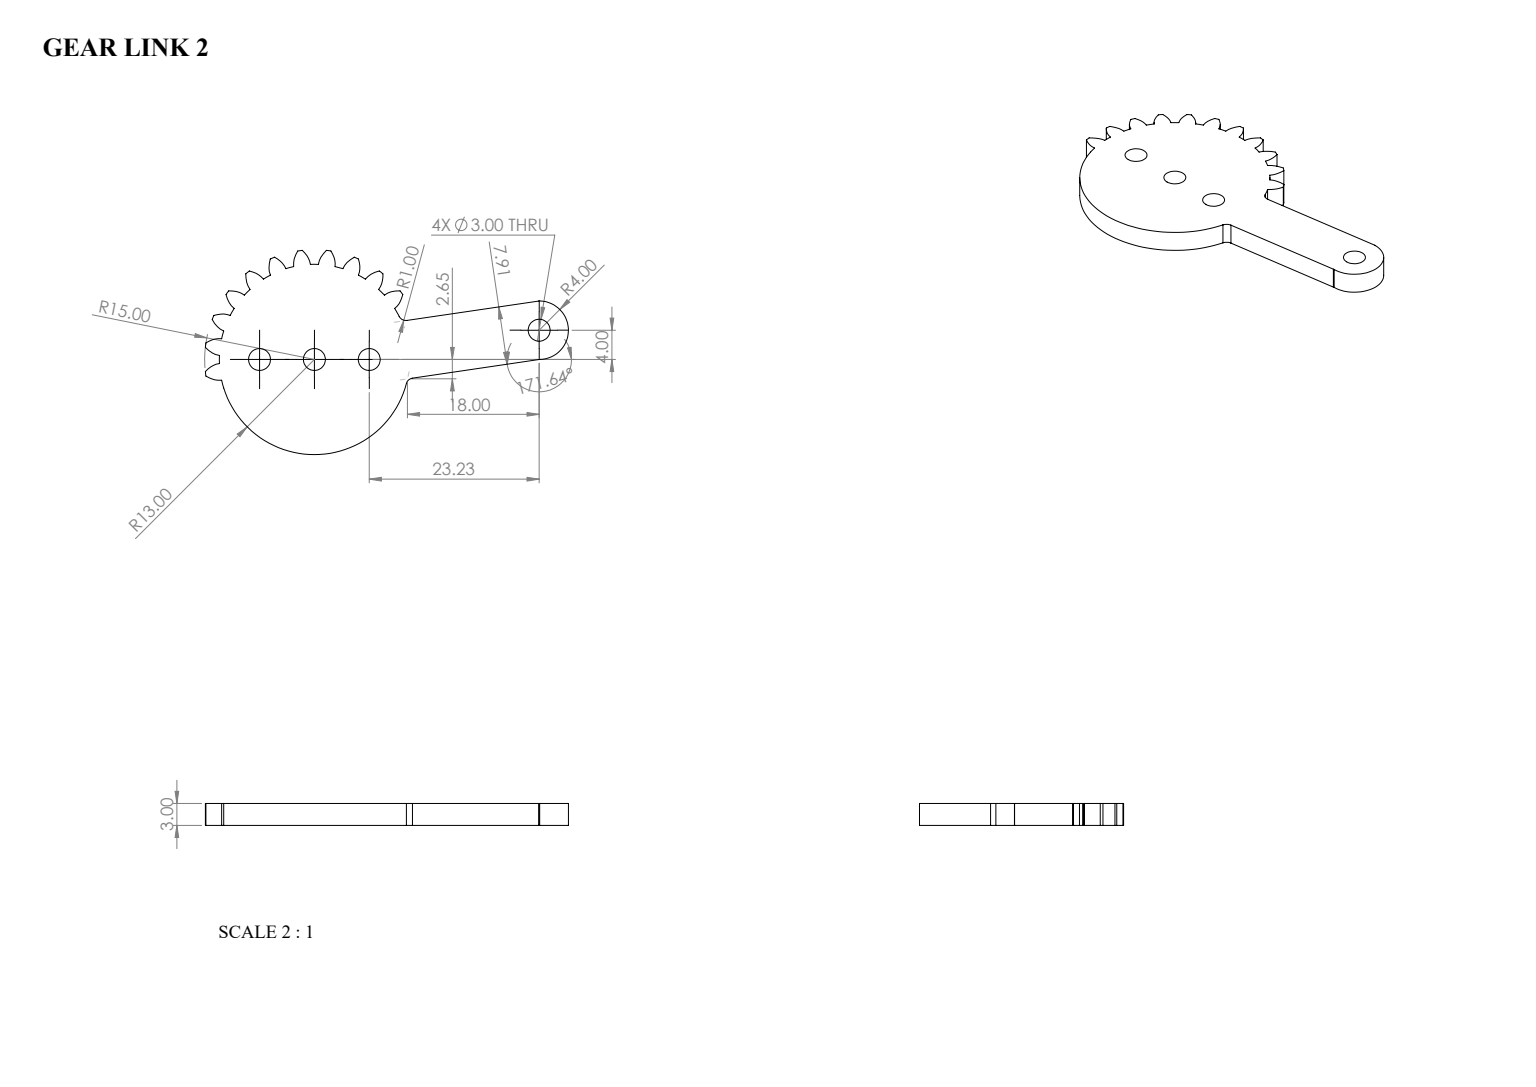
ISO-10303-21;
HEADER;
FILE_DESCRIPTION (('STEP AP214'),
    '1' );
FILE_NAME ('gear-link-2.step',
    '2026-10-11T23:18:24',
    ( '' ),
    ( '' ),
    'SwSTEP 2.0',
    'SolidWorks 2021',
    '' );
FILE_SCHEMA (( 'AUTOMOTIVE_DESIGN' ));
ENDSEC;

DATA;
#1=DIRECTION ( 'NONE',  ( 0.000000000000000000, 0.000000000000000000, -1.000000000000000000 ) ) ;
#3=ORIENTED_EDGE ( 'NONE', *, *, #624, .T. ) ;
#4=ORIENTED_EDGE ( 'NONE', *, *, #10369, .T. ) ;
#28=DIRECTION ( 'NONE',  ( 0.000000000000000000, 1.000000000000000000, 0.000000000000000000 ) ) ;
#34=CARTESIAN_POINT ( 'NONE',  ( 6.660877044263387781, 3.000000000000000000, -11.16999893002129696 ) ) ;
#42=EDGE_LOOP ( 'NONE', ( #11575, #10640, #9047, #10732 ) ) ;
#49=EDGE_CURVE ( 'NONE', #1339, #3948, #9205, .T. ) ;
#52=B_SPLINE_CURVE_WITH_KNOTS ( 'NONE', 3,
 ( #4525, #5550, #8714, #7882 ),
 .UNSPECIFIED., .F., .F.,
 ( 4, 4 ),
 ( 0.6363612417694253232, 0.6657793188270956231 ),
 .UNSPECIFIED. ) ;
#64=DIRECTION ( 'NONE',  ( 0.000000000000000000, 1.000000000000000000, 0.000000000000000000 ) ) ;
#73=LINE ( 'NONE', #7490, #793 ) ;
#82=B_SPLINE_SURFACE_WITH_KNOTS ( 'NONE', 2, 1, ( 
 ( #10714, #1415 ),
 ( #319, #8701 ),
 ( #12978, #11750 ) ),
 .UNSPECIFIED., .F., .F., .F.,
 ( 3, 3 ),
 ( 2, 2 ),
 ( 0.000000000000000000, 1.000000000000000000 ),
 ( 0.000000000000000000, 1.000000000000000000 ),
 .UNSPECIFIED. ) ;
#96=ORIENTED_EDGE ( 'NONE', *, *, #10741, .F. ) ;
#117=VERTEX_POINT ( 'NONE', #1849 ) ;
#127=CARTESIAN_POINT ( 'NONE',  ( -13.73660796332618261, 3.000000000000000000, -6.025412986832017204 ) ) ;
#132=ORIENTED_EDGE ( 'NONE', *, *, #11466, .T. ) ;
#134=DIRECTION ( 'NONE',  ( 0.000000000000000000, 0.000000000000000000, 1.000000000000000000 ) ) ;
#137=DIRECTION ( 'NONE',  ( 0.000000000000000000, 0.000000000000000000, -1.000000000000000000 ) ) ;
#144=VERTEX_POINT ( 'NONE', #5273 ) ;
#156=CARTESIAN_POINT ( 'NONE',  ( 0.5501230721522984979, 3.000000000000000000, -12.98835496148321766 ) ) ;
#157=CARTESIAN_POINT ( 'NONE',  ( -9.573149624528719315, 0.000000000000000000, -8.795158114916407754 ) ) ;
#160=ORIENTED_EDGE ( 'NONE', *, *, #10207, .F. ) ;
#161=ORIENTED_EDGE ( 'NONE', *, *, #7234, .F. ) ;
#162=B_SPLINE_SURFACE_WITH_KNOTS ( 'NONE', 3, 1, ( 
 ( #10319, #7359 ),
 ( #1025, #5084 ),
 ( #8312, #12538 ),
 ( #2123, #4325 ) ),
 .UNSPECIFIED., .F., .F., .F.,
 ( 4, 4 ),
 ( 2, 2 ),
 ( 0.000000000000000000, 0.5855695330273008592 ),
 ( 0.000000000000000000, 1.000000000000000000 ),
 .UNSPECIFIED. ) ;
#165=B_SPLINE_CURVE_WITH_KNOTS ( 'NONE', 3,
 ( #7734, #1615, #8698, #11948 ),
 .UNSPECIFIED., .F., .F.,
 ( 4, 4 ),
 ( 0.000000000000000000, 0.5855695330273008592 ),
 .UNSPECIFIED. ) ;
#166=ORIENTED_EDGE ( 'NONE', *, *, #10741, .T. ) ;
#168=DIRECTION ( 'NONE',  ( -0.000000000000000000, -1.000000000000000000, -0.000000000000000000 ) ) ;
#171=B_SPLINE_CURVE_WITH_KNOTS ( 'NONE', 3,
 ( #9035, #3811, #13254, #8012 ),
 .UNSPECIFIED., .F., .F.,
 ( 4, 4 ),
 ( 0.09090310649439187207, 0.1203211835519651524 ),
 .UNSPECIFIED. ) ;
#173=CARTESIAN_POINT ( 'NONE',  ( -8.795158114916672432, 3.000000000000000000, -9.573149624528774382 ) ) ;
#178=ORIENTED_EDGE ( 'NONE', *, *, #12277, .T. ) ;
#192=EDGE_CURVE ( 'NONE', #3774, #5500, #7308, .T. ) ;
#196=CARTESIAN_POINT ( 'NONE',  ( 13.40069634612381044, 0.000000000000000000, 2.546644602219900300 ) ) ;
#207=CARTESIAN_POINT ( 'NONE',  ( 12.08646469655232636, 3.000000000000000000, -8.883544964652022813 ) ) ;
#213=DIRECTION ( 'NONE',  ( 0.000000000000000000, 1.000000000000000000, 0.000000000000000000 ) ) ;
#215=CARTESIAN_POINT ( 'NONE',  ( -2.264806262022998062, 0.000000000000000000, -14.82803603298499340 ) ) ;
#218=ORIENTED_EDGE ( 'NONE', *, *, #842, .T. ) ;
#219=ORIENTED_EDGE ( 'NONE', *, *, #9373, .F. ) ;
#224=EDGE_CURVE ( 'NONE', #1339, #3538, #12385, .T. ) ;
#228=CARTESIAN_POINT ( 'NONE',  ( -13.52637830886122572, 3.000000000000000000, -2.928250210355275218 ) ) ;
#232=CARTESIAN_POINT ( 'NONE',  ( 2.928250210355320959, 3.000000000000000000, -13.52637830886121506 ) ) ;
#236=CARTESIAN_POINT ( 'NONE',  ( 6.970598036433451661, 3.000000000000000000, -10.97318381393796294 ) ) ;
#249=ORIENTED_EDGE ( 'NONE', *, *, #2547, .F. ) ;
#254=AXIS2_PLACEMENT_3D ( 'NONE', #5963, #13478, #3894 ) ;
#259=CARTESIAN_POINT ( 'NONE',  ( -6.970598036433426792, 3.000000000000000000, -10.97318381393771780 ) ) ;
#263=FACE_OUTER_BOUND ( 'NONE', #2351, .T. ) ;
#269=ORIENTED_EDGE ( 'NONE', *, *, #8193, .F. ) ;
#272=EDGE_LOOP ( 'NONE', ( #9491, #3874, #11052, #3338, #8276, #2839, #644, #11022, #10546, #6323, #4126, #5305, #5722, #5484, #10567, #12738, #3922, #6142, #1219, #3241, #11942, #4726, #6997, #1679, #13263, #12542, #5199, #9334, #7477, #1094, #5617, #8851, #4788, #11957, #10551, #9765, #5855, #13484, #4229, #12910, #8520, #970, #6174, #5838, #218, #6140, #7889, #11447, #8596, #13140, #12291, #13402, #12003, #12804 ) ) ;
#273=LINE ( 'NONE', #11625, #11249 ) ;
#274=CIRCLE ( 'NONE', #4001, 1.500000000000000222 ) ;
#276=B_SPLINE_SURFACE_WITH_KNOTS ( 'NONE', 3, 1, ( 
 ( #10127, #2687 ),
 ( #3651, #10063 ),
 ( #632, #13233 ),
 ( #12213, #10958 ) ),
 .UNSPECIFIED., .F., .F., .F.,
 ( 4, 4 ),
 ( 2, 2 ),
 ( 0.000000000000000000, 0.5855695330273008592 ),
 ( 0.000000000000000000, 1.000000000000000000 ),
 .UNSPECIFIED. ) ;
#281=CARTESIAN_POINT ( 'NONE',  ( 5.452638258930520010, 3.000000000000000000, -13.97385902380752754 ) ) ;
#288=VERTEX_POINT ( 'NONE', #5039 ) ;
#298=DIRECTION ( 'NONE',  ( -0.000000000000000000, -1.000000000000000000, -0.000000000000000000 ) ) ;
#300=FACE_BOUND ( 'NONE', #2086, .T. ) ;
#305=ORIENTED_EDGE ( 'NONE', *, *, #3885, .F. ) ;
#306=B_SPLINE_CURVE_WITH_KNOTS ( 'NONE', 3,
 ( #11706, #6473, #8390, #12616 ),
 .UNSPECIFIED., .F., .F.,
 ( 4, 4 ),
 ( 0.000000000000000000, 0.5855695330273008592 ),
 .UNSPECIFIED. ) ;
#315=LINE ( 'NONE', #6769, #11331 ) ;
#317=CARTESIAN_POINT ( 'NONE',  ( 1.650143266773734796, 0.000000000000000000, -14.90895795148410841 ) ) ;
#319=CARTESIAN_POINT ( 'NONE',  ( 5.741477348071313713, 3.000000000000000000, -13.86115248177180703 ) ) ;
#337=DIRECTION ( 'NONE',  ( -0.000000000000000000, -1.000000000000000000, -0.000000000000000000 ) ) ;
#360=LINE ( 'NONE', #3375, #1597 ) ;
#376=B_SPLINE_CURVE_WITH_KNOTS ( 'NONE', 2,
 ( #858, #13396, #4783 ),
 .UNSPECIFIED., .F., .F.,
 ( 3, 3 ),
 ( 0.000000000000000000, 1.000000000000000000 ),
 .UNSPECIFIED. ) ;
#385=ORIENTED_EDGE ( 'NONE', *, *, #12086, .T. ) ;
#390=CARTESIAN_POINT ( 'NONE',  ( 7.494008246337245716, 3.000000000000000000, -11.63517940784380578 ) ) ;
#391=CARTESIAN_POINT ( 'NONE',  ( -14.90895795148409420, 0.000000000000000000, 1.650143266773909101 ) ) ;
#395=CARTESIAN_POINT ( 'NONE',  ( -8.180229652970899323, 3.000000000000000000, -11.90209577080756276 ) ) ;
#406=B_SPLINE_CURVE_WITH_KNOTS ( 'NONE', 3,
 ( #3245, #11729, #7457, #5514 ),
 .UNSPECIFIED., .F., .F.,
 ( 4, 4 ),
 ( 0.1818127957067485756, 0.2112308727645026418 ),
 .UNSPECIFIED. ) ;
#411=DIRECTION ( 'NONE',  ( -0.000000000000000000, -1.000000000000000000, -0.000000000000000000 ) ) ;
#418=AXIS2_PLACEMENT_3D ( 'NONE', #13510, #5924, #10269 ) ;
#419=CARTESIAN_POINT ( 'NONE',  ( -14.90895795148411374, 0.000000000000000000, -1.650143266773683726 ) ) ;
#422=CARTESIAN_POINT ( 'NONE',  ( -5.452638258930639914, 3.000000000000000000, -13.97385902380748313 ) ) ;
#423=CARTESIAN_POINT ( 'NONE',  ( -13.52637830886122572, 0.000000000000000000, -2.928250210355275218 ) ) ;
#426=FACE_OUTER_BOUND ( 'NONE', #10907, .T. ) ;
#429=ADVANCED_FACE ( 'NONE', ( #4581 ), #2651, .F. ) ;
#430=ORIENTED_EDGE ( 'NONE', *, *, #1575, .F. ) ;
#438=CARTESIAN_POINT ( 'NONE',  ( 12.63269908545826503, 0.000000000000000000, -5.340493616518843467 ) ) ;
#448=EDGE_CURVE ( 'NONE', #3825, #117, #4011, .T. ) ;
#449=ORIENTED_EDGE ( 'NONE', *, *, #5832, .F. ) ;
#461=LINE ( 'NONE', #5837, #521 ) ;
#468=CARTESIAN_POINT ( 'NONE',  ( -0.1834773636644435324, 0.000000000000000000, -13.00394737445024873 ) ) ;
#473=CARTESIAN_POINT ( 'NONE',  ( 6.017756925049591921, 3.000000000000000000, -11.52330688609011844 ) ) ;
#483=CARTESIAN_POINT ( 'NONE',  ( -13.00394681030572208, 3.000000000000000000, -0.1834665838397169235 ) ) ;
#492=CARTESIAN_POINT ( 'NONE',  ( -2.830255545554292151, 3.000000000000000000, -12.68816982652971959 ) ) ;
#499=B_SPLINE_SURFACE_WITH_KNOTS ( 'NONE', 3, 1, ( 
 ( #6298, #5461 ),
 ( #3400, #5208 ),
 ( #10510, #11814 ),
 ( #1268, #10711 ) ),
 .UNSPECIFIED., .F., .F., .F.,
 ( 4, 4 ),
 ( 2, 2 ),
 ( 0.000000000000000000, 0.5855695330273008592 ),
 ( 0.000000000000000000, 1.000000000000000000 ),
 .UNSPECIFIED. ) ;
#501=ORIENTED_EDGE ( 'NONE', *, *, #4582, .F. ) ;
#502=ORIENTED_EDGE ( 'NONE', *, *, #9169, .T. ) ;
#511=CARTESIAN_POINT ( 'NONE',  ( -0.5501230721523990841, 0.000000000000000000, -12.98835496148299384 ) ) ;
#513=CARTESIAN_POINT ( 'NONE',  ( 8.883544964651964193, 3.000000000000000000, -12.08646469655236544 ) ) ;
#516=AXIS2_PLACEMENT_3D ( 'NONE', #8094, #8227, #869 ) ;
#520=ADVANCED_FACE ( 'NONE', ( #5381 ), #8916, .F. ) ;
#521=VECTOR ( 'NONE', #5626, 1000.000000000000000 ) ;
#522=B_SPLINE_CURVE_WITH_KNOTS ( 'NONE', 3,
 ( #12540, #2883, #11494, #4182 ),
 .UNSPECIFIED., .F., .F.,
 ( 4, 4 ),
 ( 0.000000000000000000, 0.5855695330273008592 ),
 .UNSPECIFIED. ) ;
#524=ORIENTED_EDGE ( 'NONE', *, *, #7234, .T. ) ;
#536=CARTESIAN_POINT ( 'NONE',  ( -11.90209577080766046, 3.000000000000000000, -8.180229652970757215 ) ) ;
#551=DIRECTION ( 'NONE',  ( -0.000000000000000000, -1.000000000000000000, -0.000000000000000000 ) ) ;
#556=CARTESIAN_POINT ( 'NONE',  ( -6.025412986832177076, 3.000000000000000000, -13.73660796332610268 ) ) ;
#557=ORIENTED_EDGE ( 'NONE', *, *, #3167, .F. ) ;
#565=EDGE_CURVE ( 'NONE', #13387, #8347, #11519, .T. ) ;
#567=ADVANCED_FACE ( 'NONE', ( #10952 ), #5726, .F. ) ;
#568=CARTESIAN_POINT ( 'NONE',  ( -11.52330688609014686, 0.000000000000000000, -6.017756925049552841 ) ) ;
#580=ORIENTED_EDGE ( 'NONE', *, *, #11985, .T. ) ;
#592=CARTESIAN_POINT ( 'NONE',  ( -3.893011711613112880, 0.000000000000000000, -12.40340517008282717 ) ) ;
#604=CARTESIAN_POINT ( 'NONE',  ( -12.68816982652970893, 3.000000000000000000, 2.830255545554337004 ) ) ;
#606=EDGE_LOOP ( 'NONE', ( #10674, #7647, #5644, #642 ) ) ;
#618=CARTESIAN_POINT ( 'NONE',  ( 13.40069634612381044, 3.000000000000000000, 2.546644602219900300 ) ) ;
#622=EDGE_LOOP ( 'NONE', ( #11651, #11442, #4299, #11608 ) ) ;
#623=LINE ( 'NONE', #3704, #12180 ) ;
#624=EDGE_CURVE ( 'NONE', #2462, #5247, #6615, .T. ) ;
#629=CARTESIAN_POINT ( 'NONE',  ( 12.08646469655232636, 3.000000000000000000, -8.883544964652022813 ) ) ;
#632=CARTESIAN_POINT ( 'NONE',  ( -6.329356821613726147, 3.000000000000000000, -12.30759122142001338 ) ) ;
#637=ORIENTED_EDGE ( 'NONE', *, *, #10382, .F. ) ;
#642=ORIENTED_EDGE ( 'NONE', *, *, #49, .T. ) ;
#644=ORIENTED_EDGE ( 'NONE', *, *, #13323, .T. ) ;
#670=ORIENTED_EDGE ( 'NONE', *, *, #4159, .T. ) ;
#678=EDGE_CURVE ( 'NONE', #6263, #3116, #360, .T. ) ;
#693=CARTESIAN_POINT ( 'NONE',  ( 6.329356821613516537, 3.000000000000000000, -12.30759122141987305 ) ) ;
#695=CARTESIAN_POINT ( 'NONE',  ( 3.893011711613070691, 0.000000000000000000, -12.40340517008307231 ) ) ;
#696=AXIS2_PLACEMENT_3D ( 'NONE', #10163, #9957, #13351 ) ;
#699=CARTESIAN_POINT ( 'NONE',  ( 30.82048254704846713, 0.000000000000000000, -7.998976482636475538 ) ) ;
#700=ADVANCED_FACE ( 'NONE', ( #10889 ), #9711, .F. ) ;
#701=LINE ( 'NONE', #3093, #9681 ) ;
#712=ORIENTED_EDGE ( 'NONE', *, *, #9478, .F. ) ;
#717=VECTOR ( 'NONE', #10109, 1000.000000000000000 ) ;
#721=CARTESIAN_POINT ( 'NONE',  ( -0.6724118135763151871, 0.000000000000000000, -13.82336506795071784 ) ) ;
#730=VECTOR ( 'NONE', #11828, 1000.000000000000000 ) ;
#746=VERTEX_POINT ( 'NONE', #7028 ) ;
#757=CARTESIAN_POINT ( 'NONE',  ( -11.70905276178463872, 3.000000000000000000, -9.375397774054366806 ) ) ;
#763=DIRECTION ( 'NONE',  ( 0.000000000000000000, 1.000000000000000000, 0.000000000000000000 ) ) ;
#772=AXIS2_PLACEMENT_3D ( 'NONE', #3729, #8758, #5667 ) ;
#776=CARTESIAN_POINT ( 'NONE',  ( -13.52637830886139092, 3.000000000000000000, 2.928250210355532790 ) ) ;
#777=( NAMED_UNIT ( * ) SI_UNIT ( $, .STERADIAN. ) SOLID_ANGLE_UNIT ( ) );
#786=EDGE_LOOP ( 'NONE', ( #2481, #7986, #11590, #10506 ) ) ;
#793=VECTOR ( 'NONE', #337, 1000.000000000000000 ) ;
#801=CARTESIAN_POINT ( 'NONE',  ( 10.97318381393774089, 3.000000000000000000, -6.970598036433387712 ) ) ;
#809=CARTESIAN_POINT ( 'NONE',  ( 30.73000000000000043, 0.000000000000000000, -3.999999999999999112 ) ) ;
#815=CARTESIAN_POINT ( 'NONE',  ( 0.000000000000000000, 3.000000000000000000, 0.000000000000000000 ) ) ;
#816=VERTEX_POINT ( 'NONE', #4965 ) ;
#819=ORIENTED_EDGE ( 'NONE', *, *, #11292, .T. ) ;
#827=CARTESIAN_POINT ( 'NONE',  ( -12.51336114795298471, 3.000000000000000000, -3.542894103880322998 ) ) ;
#836=B_SPLINE_CURVE_WITH_KNOTS ( 'NONE', 2,
 ( #3497, #5499, #8595 ),
 .UNSPECIFIED., .F., .F.,
 ( 3, 3 ),
 ( 0.000000000000000000, 1.000000000000000000 ),
 .UNSPECIFIED. ) ;
#838=DIRECTION ( 'NONE',  ( -0.000000000000000000, -1.000000000000000000, -0.000000000000000000 ) ) ;
#842=EDGE_CURVE ( 'NONE', #5225, #11316, #7958, .T. ) ;
#857=EDGE_CURVE ( 'NONE', #12351, #4567, #10437, .T. ) ;
#858=CARTESIAN_POINT ( 'NONE',  ( 6.025412986832064277, 0.000000000000000000, -13.73660796332615597 ) ) ;
#861=ORIENTED_EDGE ( 'NONE', *, *, #8629, .F. ) ;
#866=EDGE_CURVE ( 'NONE', #10985, #3576, #2838, .T. ) ;
#868=VERTEX_POINT ( 'NONE', #2820 ) ;
#869=DIRECTION ( 'NONE',  ( 0.000000000000000000, 0.000000000000000000, 1.000000000000000000 ) ) ;
#881=ORIENTED_EDGE ( 'NONE', *, *, #4007, .F. ) ;
#888=EDGE_CURVE ( 'NONE', #7605, #5310, #5227, .T. ) ;
#891=DIRECTION ( 'NONE',  ( -0.000000000000000000, -1.000000000000000000, -0.000000000000000000 ) ) ;
#899=VERTEX_POINT ( 'NONE', #2965 ) ;
#908=CARTESIAN_POINT ( 'NONE',  ( -13.97385902380755240, 0.000000000000000000, -5.452638258930474713 ) ) ;
#913=CARTESIAN_POINT ( 'NONE',  ( -4.821006024661084410, 3.000000000000000000, -13.61374091949017640 ) ) ;
#916=VERTEX_POINT ( 'NONE', #13435 ) ;
#926=DIRECTION ( 'NONE',  ( 0.000000000000000000, 0.000000000000000000, -1.000000000000000000 ) ) ;
#935=EDGE_CURVE ( 'NONE', #2130, #9763, #2355, .T. ) ;
#938=CARTESIAN_POINT ( 'NONE',  ( -11.90284147956865723, 0.000000000000000000, -9.133371500908332052 ) ) ;
#942=VECTOR ( 'NONE', #5646, 1000.000000000000000 ) ;
#953=VECTOR ( 'NONE', #5138, 1000.000000000000000 ) ;
#961=DIRECTION ( 'NONE',  ( -0.000000000000000000, -1.000000000000000000, -0.000000000000000000 ) ) ;
#966=ORIENTED_EDGE ( 'NONE', *, *, #7209, .T. ) ;
#970=ORIENTED_EDGE ( 'NONE', *, *, #8931, .T. ) ;
#973=CARTESIAN_POINT ( 'NONE',  ( -14.82803603298498629, 0.000000000000000000, 2.264806262023049577 ) ) ;
#974=CARTESIAN_POINT ( 'NONE',  ( 11.59535436762926430, 3.000000000000000000, -5.877734009726468756 ) ) ;
#981=AXIS2_PLACEMENT_3D ( 'NONE', #7760, #6861, #5625 ) ;
#990=CARTESIAN_POINT ( 'NONE',  ( 11.59535436762926430, 3.000000000000000000, -5.877734009726468756 ) ) ;
#999=FACE_OUTER_BOUND ( 'NONE', #9309, .T. ) ;
#1002=LINE ( 'NONE', #11939, #11502 ) ;
#1012=CARTESIAN_POINT ( 'NONE',  ( 30.65246752842885058, 3.000000000000000000, -7.988606140548566437 ) ) ;
#1014=COLOUR_RGB ( '',0.7803921568627451011, 0.7607843137254901578, 0.7411764705882353255 ) ;
#1015=EDGE_CURVE ( 'NONE', #1814, #11917, #3181, .T. ) ;
#1019=ORIENTED_EDGE ( 'NONE', *, *, #13582, .T. ) ;
#1025=CARTESIAN_POINT ( 'NONE',  ( 10.98198414889934682, 3.000000000000000000, -9.379342464487748998 ) ) ;
#1027=CARTESIAN_POINT ( 'NONE',  ( -11.52330688609014686, 0.000000000000000000, -6.017756925049552841 ) ) ;
#1029=EDGE_LOOP ( 'NONE', ( #6359, #8832, #10154, #3644 ) ) ;
#1031=ORIENTED_EDGE ( 'NONE', *, *, #12543, .T. ) ;
#1032=CARTESIAN_POINT ( 'NONE',  ( 0.1834774187694905023, 0.000000000000000000, -13.00394734430440025 ) ) ;
#1039=CARTESIAN_POINT ( 'NONE',  ( -9.379342464487789854, 3.000000000000000000, -10.98198414889931307 ) ) ;
#1040=B_SPLINE_CURVE_WITH_KNOTS ( 'NONE', 3,
 ( #2636, #10227, #3879, #8086 ),
 .UNSPECIFIED., .F., .F.,
 ( 4, 4 ),
 ( 0.000000000000000000, 0.5855695330273008592 ),
 .UNSPECIFIED. ) ;
#1048=CARTESIAN_POINT ( 'NONE',  ( -5.741477348071430065, 3.000000000000000000, -13.86115248177175374 ) ) ;
#1051=CARTESIAN_POINT ( 'NONE',  ( 1.133238802859644956, 3.000000000000000000, -14.39763212228013600 ) ) ;
#1069=CARTESIAN_POINT ( 'NONE',  ( -13.82336506795071607, 3.000000000000000000, 0.6724118135763649251 ) ) ;
#1083=CARTESIAN_POINT ( 'NONE',  ( 8.180229652970799847, 3.000000000000000000, -11.90209577080762848 ) ) ;
#1094=ORIENTED_EDGE ( 'NONE', *, *, #10459, .T. ) ;
#1099=CARTESIAN_POINT ( 'NONE',  ( 6.329356821613516537, 0.000000000000000000, -12.30759122141987305 ) ) ;
#1100=DIRECTION ( 'NONE',  ( 0.000000000000000000, 0.000000000000000000, 1.000000000000000000 ) ) ;
#1110=VERTEX_POINT ( 'NONE', #5486 ) ;
#1117=CARTESIAN_POINT ( 'NONE',  ( 30.66173999750687784, 0.000000000000000000, 0.01003121477750366919 ) ) ;
#1138=CARTESIAN_POINT ( 'NONE',  ( 11.70905276178455878, 3.000000000000000000, -9.375397774054460953 ) ) ;
#1140=CARTESIAN_POINT ( 'NONE',  ( 30.73000000000000043, 0.000000000000000000, -5.500000000000003553 ) ) ;
#1147=B_SPLINE_SURFACE_WITH_KNOTS ( 'NONE', 3, 1, ( 
 ( #8479, #9446 ),
 ( #12633, #11726 ),
 ( #8604, #11597 ),
 ( #6215, #2286 ) ),
 .UNSPECIFIED., .F., .F., .F.,
 ( 4, 4 ),
 ( 2, 2 ),
 ( 0.9090903094065657664, 0.9385083864668765097 ),
 ( 0.000000000000000000, 1.000000000000000000 ),
 .UNSPECIFIED. ) ;
#1157=DIRECTION ( 'NONE',  ( 0.000000000000000000, 1.000000000000000000, -0.000000000000000000 ) ) ;
#1173=CARTESIAN_POINT ( 'NONE',  ( -1.650143266773857142, 0.000000000000000000, -14.90895795148409952 ) ) ;
#1176=B_SPLINE_CURVE_WITH_KNOTS ( 'NONE', 3,
 ( #9855, #7659, #4562, #9597 ),
 .UNSPECIFIED., .F., .F.,
 ( 4, 4 ),
 ( 0.000000000000000000, 0.5855695330273008592 ),
 .UNSPECIFIED. ) ;
#1188=AXIS2_PLACEMENT_3D ( 'NONE', #809, #5000, #9194 ) ;
#1190=CARTESIAN_POINT ( 'NONE',  ( 9.299128225235451239, 3.000000000000000000, -10.25006213149493561 ) ) ;
#1195=LINE ( 'NONE', #173, #5307 ) ;
#1197=ORIENTED_EDGE ( 'NONE', *, *, #4427, .T. ) ;
#1206=ADVANCED_FACE ( 'NONE', ( #5426 ), #6831, .F. ) ;
#1214=CARTESIAN_POINT ( 'NONE',  ( 6.025412986832064277, 3.000000000000000000, -13.73660796332615597 ) ) ;
#1219=ORIENTED_EDGE ( 'NONE', *, *, #12818, .T. ) ;
#1221=ADVANCED_FACE ( 'NONE', ( #13141 ), #3750, .F. ) ;
#1228=CARTESIAN_POINT ( 'NONE',  ( -7.500000000000000000, 0.000000000000000000, 0.000000000000000000 ) ) ;
#1233=ORIENTED_EDGE ( 'NONE', *, *, #4398, .F. ) ;
#1238=CARTESIAN_POINT ( 'NONE',  ( 13.54609072798131209, 3.000000000000000000, 3.536018380791111415 ) ) ;
#1239=SURFACE_SIDE_STYLE ('',( #2602 ) ) ;
#1242=CARTESIAN_POINT ( 'NONE',  ( -1.958311002203252160, 3.000000000000000000, -14.87484884897975768 ) ) ;
#1245=ORIENTED_EDGE ( 'NONE', *, *, #13083, .F. ) ;
#1258=PLANE ( 'NONE',  #10858 ) ;
#1268=CARTESIAN_POINT ( 'NONE',  ( 6.025412986832064277, 3.000000000000000000, -13.73660796332615597 ) ) ;
#1269=EDGE_CURVE ( 'NONE', #9570, #11420, #3803, .T. ) ;
#1271=CARTESIAN_POINT ( 'NONE',  ( 1.133238802859644956, 0.000000000000000000, -14.39763212228013600 ) ) ;
#1272=CARTESIAN_POINT ( 'NONE',  ( -9.324917476840782982, 0.000000000000000000, -9.065441278446241924 ) ) ;
#1285=CARTESIAN_POINT ( 'NONE',  ( -6.660869762029062890, 3.000000000000000000, -11.17001010193236610 ) ) ;
#1286=B_SPLINE_CURVE_WITH_KNOTS ( 'NONE', 2,
 ( #7443, #4476, #6606 ),
 .UNSPECIFIED., .F., .F.,
 ( 3, 3 ),
 ( 0.000000000000000000, 1.000000000000000000 ),
 .UNSPECIFIED. ) ;
#1288=EDGE_CURVE ( 'NONE', #11402, #5247, #1374, .T. ) ;
#1300=LINE ( 'NONE', #2341, #8363 ) ;
#1305=CARTESIAN_POINT ( 'NONE',  ( -13.17831234185052836, 3.000000000000000000, -4.227250083625696320 ) ) ;
#1308=EDGE_LOOP ( 'NONE', ( #1538, #9293, #4547, #5125 ) ) ;
#1309=ORIENTED_EDGE ( 'NONE', *, *, #2939, .F. ) ;
#1310=CIRCLE ( 'NONE', #1531, 1.000000000000001776 ) ;
#1314=B_SPLINE_CURVE_WITH_KNOTS ( 'NONE', 2,
 ( #391, #12036, #6720 ),
 .UNSPECIFIED., .F., .F.,
 ( 3, 3 ),
 ( 0.000000000000000000, 1.000000000000000000 ),
 .UNSPECIFIED. ) ;
#1322=CARTESIAN_POINT ( 'NONE',  ( -7.500000000000000000, 3.000000000000000000, 1.500000000000000666 ) ) ;
#1326=ORIENTED_EDGE ( 'NONE', *, *, #3867, .F. ) ;
#1339=VERTEX_POINT ( 'NONE', #4111 ) ;
#1346=B_SPLINE_CURVE_WITH_KNOTS ( 'NONE', 3,
 ( #695, #4888, #9088, #13305 ),
 .UNSPECIFIED., .F., .F.,
 ( 4, 4 ),
 ( 0.7272709309819391787, 0.7566890080396341256 ),
 .UNSPECIFIED. ) ;
#1355=VECTOR ( 'NONE', #2270, 1000.000000000000000 ) ;
#1356=CARTESIAN_POINT ( 'NONE',  ( 2.631756770590782057, 0.000000000000000000, -14.20034848914875347 ) ) ;
#1359=EDGE_CURVE ( 'NONE', #11340, #1456, #10893, .T. ) ;
#1366=EDGE_CURVE ( 'NONE', #11919, #2149, #5640, .T. ) ;
#1369=FILL_AREA_STYLE_COLOUR ( '', #1014 ) ;
#1370=B_SPLINE_SURFACE_WITH_KNOTS ( 'NONE', 3, 1, ( 
 ( #5624, #9822 ),
 ( #536, #4591 ),
 ( #12042, #8847 ),
 ( #8776, #13068 ) ),
 .UNSPECIFIED., .F., .F., .F.,
 ( 4, 4 ),
 ( 2, 2 ),
 ( 0.000000000000000000, 0.5855695330273008592 ),
 ( 0.000000000000000000, 1.000000000000000000 ),
 .UNSPECIFIED. ) ;
#1374=B_SPLINE_CURVE_WITH_KNOTS ( 'NONE', 2,
 ( #2805, #7013, #1778 ),
 .UNSPECIFIED., .F., .F.,
 ( 3, 3 ),
 ( 0.000000000000000000, 1.000000000000000000 ),
 .UNSPECIFIED. ) ;
#1376=ORIENTED_EDGE ( 'NONE', *, *, #4336, .T. ) ;
#1382=ORIENTED_EDGE ( 'NONE', *, *, #1952, .F. ) ;
#1385=B_SPLINE_CURVE_WITH_KNOTS ( 'NONE', 3,
 ( #4618, #8805, #3586, #7305 ),
 .UNSPECIFIED., .F., .F.,
 ( 4, 4 ),
 ( 0.000000000000000000, 0.5855695330273008592 ),
 .UNSPECIFIED. ) ;
#1387=ORIENTED_EDGE ( 'NONE', *, *, #4398, .T. ) ;
#1388=CARTESIAN_POINT ( 'NONE',  ( -12.98835496148321944, 3.000000000000000000, -0.5501230721522550882 ) ) ;
#1393=CARTESIAN_POINT ( 'NONE',  ( -12.68816982652953840, 3.000000000000000000, -2.830255545554093644 ) ) ;
#1415=CARTESIAN_POINT ( 'NONE',  ( 6.025412986832064277, 0.000000000000000000, -13.73660796332615597 ) ) ;
#1416=DIRECTION ( 'NONE',  ( -0.000000000000000000, -1.000000000000000000, -0.000000000000000000 ) ) ;
#1428=CARTESIAN_POINT ( 'NONE',  ( 30.79786191028635400, 3.000000000000000000, -7.999232361977356653 ) ) ;
#1433=FACE_OUTER_BOUND ( 'NONE', #9405, .T. ) ;
#1436=ORIENTED_EDGE ( 'NONE', *, *, #1948, .F. ) ;
#1439=ORIENTED_EDGE ( 'NONE', *, *, #8319, .F. ) ;
#1441=VERTEX_POINT ( 'NONE', #1624 ) ;
#1456=VERTEX_POINT ( 'NONE', #592 ) ;
#1467=FACE_BOUND ( 'NONE', #10598, .T. ) ;
#1468=CARTESIAN_POINT ( 'NONE',  ( -12.68816982652953840, 3.000000000000000000, -2.830255545554093644 ) ) ;
#1480=CARTESIAN_POINT ( 'NONE',  ( 0.5501230721522984979, 0.000000000000000000, -12.98835496148321766 ) ) ;
#1486=B_SPLINE_SURFACE_WITH_KNOTS ( 'NONE', 3, 1, ( 
 ( #8264, #973 ),
 ( #9432, #4193 ),
 ( #776, #4969 ),
 ( #13377, #9164 ) ),
 .UNSPECIFIED., .F., .F., .F.,
 ( 4, 4 ),
 ( 2, 2 ),
 ( 0.000000000000000000, 0.5855695330273008592 ),
 ( 0.000000000000000000, 1.000000000000000000 ),
 .UNSPECIFIED. ) ;
#1504=EDGE_LOOP ( 'NONE', ( #1890, #2339, #249, #3 ) ) ;
#1517=CARTESIAN_POINT ( 'NONE',  ( -13.00394681030572208, 0.000000000000000000, -0.1834665838397169235 ) ) ;
#1524=B_SPLINE_CURVE_WITH_KNOTS ( 'NONE', 3,
 ( #12864, #7682, #390, #9619 ),
 .UNSPECIFIED., .F., .F.,
 ( 4, 4 ),
 ( 0.000000000000000000, 0.5855695330273008592 ),
 .UNSPECIFIED. ) ;
#1529=CARTESIAN_POINT ( 'NONE',  ( 9.065480927540312095, 0.000000000000000000, -9.324856600128422102 ) ) ;
#1531=AXIS2_PLACEMENT_3D ( 'NONE', #1238, #4264, #5428 ) ;
#1533=ORIENTED_EDGE ( 'NONE', *, *, #12497, .F. ) ;
#1536=VERTEX_POINT ( 'NONE', #7032 ) ;
#1537=EDGE_CURVE ( 'NONE', #13428, #13474, #4113, .T. ) ;
#1538=ORIENTED_EDGE ( 'NONE', *, *, #12078, .T. ) ;
#1553=ORIENTED_EDGE ( 'NONE', *, *, #10207, .T. ) ;
#1558=CARTESIAN_POINT ( 'NONE',  ( -1.650143266773857142, 0.000000000000000000, -14.90895795148409952 ) ) ;
#1566=CARTESIAN_POINT ( 'NONE',  ( -13.61374091949023679, 3.000000000000000000, -4.821006024660923650 ) ) ;
#1568=AXIS2_PLACEMENT_3D ( 'NONE', #12469, #12655, #8432 ) ;
#1570=ORIENTED_EDGE ( 'NONE', *, *, #2217, .F. ) ;
#1575=EDGE_CURVE ( 'NONE', #6867, #8751, #9965, .T. ) ;
#1582=FACE_OUTER_BOUND ( 'NONE', #2814, .T. ) ;
#1593=FACE_OUTER_BOUND ( 'NONE', #5258, .T. ) ;
#1597=VECTOR ( 'NONE', #7587, 1000.000000000000000 ) ;
#1608=VERTEX_POINT ( 'NONE', #10196 ) ;
#1609=ORIENTED_EDGE ( 'NONE', *, *, #2578, .F. ) ;
#1615=CARTESIAN_POINT ( 'NONE',  ( 10.98198414889934682, 0.000000000000000000, -9.379342464487748998 ) ) ;
#1619=CARTESIAN_POINT ( 'NONE',  ( -9.065441275458884007, 0.000000000000000000, -9.324917484779556176 ) ) ;
#1623=VECTOR ( 'NONE', #2118, 1000.000000000000000 ) ;
#1624=CARTESIAN_POINT ( 'NONE',  ( 8.795158114916441505, 3.000000000000000000, -9.573149624528689117 ) ) ;
#1627=AXIS2_PLACEMENT_3D ( 'NONE', #11632, #9626, #8578 ) ;
#1638=EDGE_CURVE ( 'NONE', #12749, #2659, #1346, .T. ) ;
#1640=CARTESIAN_POINT ( 'NONE',  ( -2.830255545554292151, 3.000000000000000000, -12.68816982652971959 ) ) ;
#1648=EDGE_LOOP ( 'NONE', ( #5645, #712, #3236, #11092 ) ) ;
#1651=VERTEX_POINT ( 'NONE', #9558 ) ;
#1654=VECTOR ( 'NONE', #5931, 1000.000000000000000 ) ;
#1661=ORIENTED_EDGE ( 'NONE', *, *, #2538, .F. ) ;
#1679=ORIENTED_EDGE ( 'NONE', *, *, #5232, .T. ) ;
#1680=ORIENTED_EDGE ( 'NONE', *, *, #6158, .F. ) ;
#1693=CARTESIAN_POINT ( 'NONE',  ( -3.893011711613112880, 3.000000000000000000, -12.40340517008282717 ) ) ;
#1695=DIRECTION ( 'NONE',  ( 0.000000000000000000, 1.000000000000000000, -0.000000000000000000 ) ) ;
#1696=ORIENTED_EDGE ( 'NONE', *, *, #4159, .F. ) ;
#1702=CARTESIAN_POINT ( 'NONE',  ( -6.970598036433426792, 0.000000000000000000, -10.97318381393771780 ) ) ;
#1705=ADVANCED_FACE ( 'NONE', ( #8638 ), #3873, .F. ) ;
#1716=EDGE_CURVE ( 'NONE', #8003, #11262, #1524, .T. ) ;
#1718=DIRECTION ( 'NONE',  ( -0.000000000000000000, -1.000000000000000000, -0.000000000000000000 ) ) ;
#1722=CARTESIAN_POINT ( 'NONE',  ( -14.90895795148411374, 3.000000000000000000, -1.650143266773683726 ) ) ;
#1726=ORIENTED_EDGE ( 'NONE', *, *, #7893, .F. ) ;
#1731=CARTESIAN_POINT ( 'NONE',  ( 6.025412986832064277, 3.000000000000000000, -13.73660796332615597 ) ) ;
#1741=CARTESIAN_POINT ( 'NONE',  ( -12.40340517008309185, 3.000000000000000000, -3.893011711613028947 ) ) ;
#1748=ORIENTED_EDGE ( 'NONE', *, *, #9633, .T. ) ;
#1749=CARTESIAN_POINT ( 'NONE',  ( -6.025412986832177076, 3.000000000000000000, -13.73660796332610268 ) ) ;
#1751=CARTESIAN_POINT ( 'NONE',  ( -7.494008246337227952, 0.000000000000000000, -11.63517940784355886 ) ) ;
#1762=ORIENTED_EDGE ( 'NONE', *, *, #13322, .F. ) ;
#1769=CARTESIAN_POINT ( 'NONE',  ( 6.343080161942737938, 0.000000000000000000, -11.35348358516942469 ) ) ;
#1771=CARTESIAN_POINT ( 'NONE',  ( -14.82803603298498629, 3.000000000000000000, 2.264806262023049577 ) ) ;
#1772=ADVANCED_FACE ( 'NONE', ( #5348 ), #4522, .F. ) ;
#1778=CARTESIAN_POINT ( 'NONE',  ( 1.650143266773734796, 0.000000000000000000, -14.90895795148410841 ) ) ;
#1787=VECTOR ( 'NONE', #5884, 1000.000000000000000 ) ;
#1795=ORIENTED_EDGE ( 'NONE', *, *, #6353, .F. ) ;
#1814=VERTEX_POINT ( 'NONE', #1558 ) ;
#1822=VECTOR ( 'NONE', #2673, 1000.000000000000000 ) ;
#1830=CARTESIAN_POINT ( 'NONE',  ( -0.6724118135763151871, 3.000000000000000000, -13.82336506795071784 ) ) ;
#1837=ORIENTED_EDGE ( 'NONE', *, *, #5832, .T. ) ;
#1842=CARTESIAN_POINT ( 'NONE',  ( -8.795158114916672432, 3.000000000000000000, -9.573149624528774382 ) ) ;
#1849=CARTESIAN_POINT ( 'NONE',  ( 12.57851281883977457, 3.000000000000000000, 3.283445639306028063 ) ) ;
#1853=EDGE_LOOP ( 'NONE', ( #6961, #4497, #1680, #7692 ) ) ;
#1854=EDGE_CURVE ( 'NONE', #6430, #6340, #12989, .T. ) ;
#1870=ORIENTED_EDGE ( 'NONE', *, *, #9876, .T. ) ;
#1883=DIRECTION ( 'NONE',  ( -0.000000000000000000, -1.000000000000000000, -0.000000000000000000 ) ) ;
#1886=VECTOR ( 'NONE', #961, 1000.000000000000000 ) ;
#1890=ORIENTED_EDGE ( 'NONE', *, *, #10284, .T. ) ;
#1894=AXIS2_PLACEMENT_3D ( 'NONE', #10392, #13498, #1 ) ;
#1895=CARTESIAN_POINT ( 'NONE',  ( 10.98198414889934682, 3.000000000000000000, -9.379342464487748998 ) ) ;
#1907=PRODUCT_DEFINITION_FORMATION_WITH_SPECIFIED_SOURCE ( 'ANY', '', #7531, .NOT_KNOWN. ) ;
#1908=ORIENTED_EDGE ( 'NONE', *, *, #8249, .T. ) ;
#1915=B_SPLINE_SURFACE_WITH_KNOTS ( 'NONE', 3, 1, ( 
 ( #3445, #568 ),
 ( #13165, #2685 ),
 ( #6890, #7654 ),
 ( #11857, #2416 ) ),
 .UNSPECIFIED., .F., .F., .F.,
 ( 4, 4 ),
 ( 2, 2 ),
 ( 0.000000000000000000, 0.5855695330273008592 ),
 ( 0.000000000000000000, 1.000000000000000000 ),
 .UNSPECIFIED. ) ;
#1916=CARTESIAN_POINT ( 'NONE',  ( -14.87484884897975057, 3.000000000000000000, 1.958311002203303453 ) ) ;
#1921=ORIENTED_EDGE ( 'NONE', *, *, #9861, .T. ) ;
#1923=CARTESIAN_POINT ( 'NONE',  ( -3.188443695493920593, 0.000000000000000000, -12.60833606734848189 ) ) ;
#1929=CARTESIAN_POINT ( 'NONE',  ( -12.60833596047604210, 0.000000000000000000, -3.188441730140805674 ) ) ;
#1939=FACE_OUTER_BOUND ( 'NONE', #12013, .T. ) ;
#1941=CARTESIAN_POINT ( 'NONE',  ( 1.650143266773734796, 0.000000000000000000, -14.90895795148410841 ) ) ;
#1948=EDGE_CURVE ( 'NONE', #3825, #916, #12465, .T. ) ;
#1952=EDGE_CURVE ( 'NONE', #12534, #13401, #6453, .T. ) ;
#1958=LINE ( 'NONE', #13534, #11523 ) ;
#1961=CARTESIAN_POINT ( 'NONE',  ( -14.90895795148409420, 3.000000000000000000, 1.650143266773909101 ) ) ;
#1970=EDGE_CURVE ( 'NONE', #3576, #11919, #6278, .T. ) ;
#1972=CARTESIAN_POINT ( 'NONE',  ( -3.188443695493920593, 3.000000000000000000, -12.60833606734848189 ) ) ;
#1974=DIRECTION ( 'NONE',  ( -0.000000000000000000, -1.000000000000000000, -0.000000000000000000 ) ) ;
#1975=LINE ( 'NONE', #1012, #7945 ) ;
#1992=CARTESIAN_POINT ( 'NONE',  ( 30.73000000000000043, 3.000000000000000000, -2.499999999999995115 ) ) ;
#2001=CYLINDRICAL_SURFACE ( 'NONE', #418, 3.999999999999997335 ) ;
#2007=FACE_OUTER_BOUND ( 'NONE', #1504, .T. ) ;
#2010=ORIENTED_EDGE ( 'NONE', *, *, #7467, .F. ) ;
#2014=CARTESIAN_POINT ( 'NONE',  ( -5.741477348071430065, 0.000000000000000000, -13.86115248177175374 ) ) ;
#2020=CARTESIAN_POINT ( 'NONE',  ( -10.97318381393799136, 0.000000000000000000, -6.970598036433411693 ) ) ;
#2025=DIRECTION ( 'NONE',  ( -0.000000000000000000, -1.000000000000000000, -0.000000000000000000 ) ) ;
#2039=ADVANCED_FACE ( 'NONE', ( #2857 ), #6234, .F. ) ;
#2043=CARTESIAN_POINT ( 'NONE',  ( 6.970598036433451661, 0.000000000000000000, -10.97318381393796294 ) ) ;
#2045=EDGE_CURVE ( 'NONE', #4765, #7515, #2995, .T. ) ;
#2069=CARTESIAN_POINT ( 'NONE',  ( -0.1834773636644435324, 0.000000000000000000, -13.00394737445024873 ) ) ;
#2070=ORIENTED_EDGE ( 'NONE', *, *, #4899, .T. ) ;
#2078=CARTESIAN_POINT ( 'NONE',  ( -12.56843238770841786, 3.000000000000000000, 3.367671042046304741 ) ) ;
#2079=CARTESIAN_POINT ( 'NONE',  ( 1.650143266773734796, 3.000000000000000000, -14.90895795148410841 ) ) ;
#2086=EDGE_LOOP ( 'NONE', ( #3854, #8076 ) ) ;
#2095=CARTESIAN_POINT ( 'NONE',  ( 12.08646469655232636, 3.000000000000000000, -8.883544964652022813 ) ) ;
#2101=EDGE_CURVE ( 'NONE', #6340, #9161, #7137, .T. ) ;
#2113=ORIENTED_EDGE ( 'NONE', *, *, #1970, .F. ) ;
#2114=EDGE_CURVE ( 'NONE', #117, #4831, #9542, .T. ) ;
#2118=DIRECTION ( 'NONE',  ( -0.000000000000000000, -1.000000000000000000, -0.000000000000000000 ) ) ;
#2123=CARTESIAN_POINT ( 'NONE',  ( 9.573149624528804580, 3.000000000000000000, -8.795158114916638681 ) ) ;
#2124=CARTESIAN_POINT ( 'NONE',  ( -12.68816982652953840, 3.000000000000000000, -2.830255545554093644 ) ) ;
#2125=CARTESIAN_POINT ( 'NONE',  ( -10.97318381393799136, 3.000000000000000000, -6.970598036433411693 ) ) ;
#2127=ADVANCED_FACE ( 'NONE', ( #11745 ), #6083, .F. ) ;
#2130=VERTEX_POINT ( 'NONE', #10710 ) ;
#2135=B_SPLINE_SURFACE_WITH_KNOTS ( 'NONE', 3, 1, ( 
 ( #4543, #6477 ),
 ( #10613, #10685 ),
 ( #1305, #9641 ),
 ( #4406, #6682 ) ),
 .UNSPECIFIED., .F., .F., .F.,
 ( 4, 4 ),
 ( 2, 2 ),
 ( 0.000000000000000000, 0.5855695330273008592 ),
 ( 0.000000000000000000, 1.000000000000000000 ),
 .UNSPECIFIED. ) ;
#2143=ORIENTED_EDGE ( 'NONE', *, *, #7450, .T. ) ;
#2146=ORIENTED_EDGE ( 'NONE', *, *, #9861, .F. ) ;
#2149=VERTEX_POINT ( 'NONE', #4303 ) ;
#2158=CARTESIAN_POINT ( 'NONE',  ( 13.54609072798131209, 3.000000000000000000, 3.536018380791111415 ) ) ;
#2162=ORIENTED_EDGE ( 'NONE', *, *, #12261, .F. ) ;
#2167=CARTESIAN_POINT ( 'NONE',  ( -14.90895795148409420, 0.000000000000000000, 1.650143266773909101 ) ) ;
#2173=B_SPLINE_CURVE_WITH_KNOTS ( 'NONE', 3,
 ( #11816, #8826, #13050, #2579 ),
 .UNSPECIFIED., .F., .F.,
 ( 4, 4 ),
 ( 0.000000000000000000, 0.5855695330273008592 ),
 .UNSPECIFIED. ) ;
#2174=DIRECTION ( 'NONE',  ( 0.000000000000000000, 1.000000000000000000, -0.000000000000000000 ) ) ;
#2179=CARTESIAN_POINT ( 'NONE',  ( -14.82803603298502360, 0.000000000000000000, -2.264806262022826644 ) ) ;
#2181=CARTESIAN_POINT ( 'NONE',  ( 7.494008246337245716, 0.000000000000000000, -11.63517940784380578 ) ) ;
#2189=ORIENTED_EDGE ( 'NONE', *, *, #12522, .F. ) ;
#2202=DIRECTION ( 'NONE',  ( 0.000000000000000000, 0.000000000000000000, 1.000000000000000000 ) ) ;
#2209=ORIENTED_EDGE ( 'NONE', *, *, #5475, .F. ) ;
#2210=CARTESIAN_POINT ( 'NONE',  ( -6.025412986832177076, 3.000000000000000000, -13.73660796332610268 ) ) ;
#2217=EDGE_CURVE ( 'NONE', #11316, #11354, #9554, .T. ) ;
#2220=CARTESIAN_POINT ( 'NONE',  ( 2.264806262022877714, 0.000000000000000000, -14.82803603298501471 ) ) ;
#2222=CARTESIAN_POINT ( 'NONE',  ( -9.573149624528719315, 3.000000000000000000, -8.795158114916407754 ) ) ;
#2234=LINE ( 'NONE', #10653, #9228 ) ;
#2235=CARTESIAN_POINT ( 'NONE',  ( -11.90284147956865723, 0.000000000000000000, -9.133371500908332052 ) ) ;
#2236=B_SPLINE_CURVE_WITH_KNOTS ( 'NONE', 3,
 ( #12874, #3419, #5556, #3153 ),
 .UNSPECIFIED., .F., .F.,
 ( 4, 4 ),
 ( 0.000000000000000000, 0.5855695330273008592 ),
 .UNSPECIFIED. ) ;
#2237=CARTESIAN_POINT ( 'NONE',  ( 30.79786191028635400, 3.000000000000000000, -6.999232361977355765 ) ) ;
#2251=CARTESIAN_POINT ( 'NONE',  ( 2.264806262022877714, 0.000000000000000000, -14.82803603298501471 ) ) ;
#2262=CARTESIAN_POINT ( 'NONE',  ( 9.573149624528804580, 3.000000000000000000, -8.795158114916638681 ) ) ;
#2267=CARTESIAN_POINT ( 'NONE',  ( 13.54609072798131209, 0.000000000000000000, 3.536018380791111415 ) ) ;
#2270=DIRECTION ( 'NONE',  ( -0.000000000000000000, -1.000000000000000000, -0.000000000000000000 ) ) ;
#2274=ORIENTED_EDGE ( 'NONE', *, *, #1537, .F. ) ;
#2281=VECTOR ( 'NONE', #9666, 1000.000000000000000 ) ;
#2284=DIRECTION ( 'NONE',  ( 0.9893737785712105604, -0.000000000000000000, -0.1453943818575020863 ) ) ;
#2286=CARTESIAN_POINT ( 'NONE',  ( 8.795158114916441505, 0.000000000000000000, -9.573149624528689117 ) ) ;
#2288=DIRECTION ( 'NONE',  ( -0.000000000000000000, -1.000000000000000000, -0.000000000000000000 ) ) ;
#2290=CARTESIAN_POINT ( 'NONE',  ( 6.343080161942737938, 3.000000000000000000, -11.35348358516942469 ) ) ;
#2296=CARTESIAN_POINT ( 'NONE',  ( 6.660877044263387781, 0.000000000000000000, -11.16999893002129696 ) ) ;
#2298=B_SPLINE_CURVE_WITH_KNOTS ( 'NONE', 3,
 ( #10242, #13270, #3829, #10304 ),
 .UNSPECIFIED., .F., .F.,
 ( 4, 4 ),
 ( 0.000000000000000000, 0.5855695330273008592 ),
 .UNSPECIFIED. ) ;
#2303=ORIENTED_EDGE ( 'NONE', *, *, #9275, .F. ) ;
#2305=B_SPLINE_CURVE_WITH_KNOTS ( 'NONE', 3,
 ( #6119, #2807, #7016, #9208 ),
 .UNSPECIFIED., .F., .F.,
 ( 4, 4 ),
 ( 0.000000000000000000, 0.5855695330273008592 ),
 .UNSPECIFIED. ) ;
#2306=CARTESIAN_POINT ( 'NONE',  ( -13.82336506795071607, 0.000000000000000000, 0.6724118135763649251 ) ) ;
#2313=CARTESIAN_POINT ( 'NONE',  ( -1.650143266773857142, 3.000000000000000000, -14.90895795148409952 ) ) ;
#2317=VECTOR ( 'NONE', #168, 1000.000000000000000 ) ;
#2318=CIRCLE ( 'NONE', #1894, 1.000000000000000888 ) ;
#2325=B_SPLINE_CURVE_WITH_KNOTS ( 'NONE', 3,
 ( #9684, #11969, #12932, #10927 ),
 .UNSPECIFIED., .F., .F.,
 ( 4, 4 ),
 ( 0.000000000000000000, 0.5855695330273008592 ),
 .UNSPECIFIED. ) ;
#2329=CARTESIAN_POINT ( 'NONE',  ( -6.343077614891082128, 3.000000000000000000, -11.35348748332310720 ) ) ;
#2330=CARTESIAN_POINT ( 'NONE',  ( -13.86115248177182835, 0.000000000000000000, -5.741477348071267528 ) ) ;
#2339=ORIENTED_EDGE ( 'NONE', *, *, #7209, .F. ) ;
#2341=CARTESIAN_POINT ( 'NONE',  ( 30.82048254704846713, 3.000000000000000000, -7.998976482636475538 ) ) ;
#2343=DIRECTION ( 'NONE',  ( 0.000000000000000000, 0.000000000000000000, -1.000000000000000000 ) ) ;
#2351=EDGE_LOOP ( 'NONE', ( #6981, #2596, #6036, #2146 ) ) ;
#2352=CARTESIAN_POINT ( 'NONE',  ( -13.00394572736061605, 0.000000000000000000, 0.1835083749157108701 ) ) ;
#2355=B_SPLINE_CURVE_WITH_KNOTS ( 'NONE', 3,
 ( #7300, #1032, #2069, #9426 ),
 .UNSPECIFIED., .F., .F.,
 ( 4, 4 ),
 ( 0.6363612417694253232, 0.6657793188270956231 ),
 .UNSPECIFIED. ) ;
#2359=CARTESIAN_POINT ( 'NONE',  ( -8.883544964652065445, 3.000000000000000000, -12.08646469655229438 ) ) ;
#2366=CARTESIAN_POINT ( 'NONE',  ( 6.343080161942737938, 0.000000000000000000, -11.35348358516942469 ) ) ;
#2376=CARTESIAN_POINT ( 'NONE',  ( -11.70905276178463872, 3.000000000000000000, -9.375397774054366806 ) ) ;
#2380=VERTEX_POINT ( 'NONE', #4010 ) ;
#2398=CARTESIAN_POINT ( 'NONE',  ( 12.08646469655232636, 0.000000000000000000, -8.883544964652022813 ) ) ;
#2401=( NAMED_UNIT ( * ) SI_UNIT ( $, .STERADIAN. ) SOLID_ANGLE_UNIT ( ) );
#2412=ORIENTED_EDGE ( 'NONE', *, *, #5232, .F. ) ;
#2413=DIRECTION ( 'NONE',  ( 0.9893737785712105604, 0.000000000000000000, -0.1453943818575021141 ) ) ;
#2416=CARTESIAN_POINT ( 'NONE',  ( -13.73660796332618261, 0.000000000000000000, -6.025412986832017204 ) ) ;
#2419=DIRECTION ( 'NONE',  ( 0.000000000000000000, 0.000000000000000000, 1.000000000000000000 ) ) ;
#2426=VERTEX_POINT ( 'NONE', #12443 ) ;
#2434=ADVANCED_BREP_SHAPE_REPRESENTATION ( '', ( #4005, #10007 ), #6949 ) ;
#2444=CARTESIAN_POINT ( 'NONE',  ( 4.821006024660968947, 3.000000000000000000, -13.61374091949021015 ) ) ;
#2448=VERTEX_POINT ( 'NONE', #1749 ) ;
#2462=VERTEX_POINT ( 'NONE', #13529 ) ;
#2470=( NAMED_UNIT ( * ) SI_UNIT ( $, .STERADIAN. ) SOLID_ANGLE_UNIT ( ) );
#2471=B_SPLINE_SURFACE_WITH_KNOTS ( 'NONE', 3, 1, ( 
 ( #8433, #8498 ),
 ( #3851, #3981 ),
 ( #8116, #11365 ),
 ( #5018, #2958 ) ),
 .UNSPECIFIED., .F., .F., .F.,
 ( 4, 4 ),
 ( 2, 2 ),
 ( 0.7272709309819391787, 0.7566890080396341256 ),
 ( 0.000000000000000000, 1.000000000000000000 ),
 .UNSPECIFIED. ) ;
#2473=CARTESIAN_POINT ( 'NONE',  ( -10.25006213149496936, 3.000000000000000000, -9.299128225235415712 ) ) ;
#2481=ORIENTED_EDGE ( 'NONE', *, *, #3216, .T. ) ;
#2483=EDGE_CURVE ( 'NONE', #3948, #9570, #10881, .T. ) ;
#2495=CARTESIAN_POINT ( 'NONE',  ( -12.68816982652970893, 0.000000000000000000, 2.830255545554337004 ) ) ;
#2498=EDGE_LOOP ( 'NONE', ( #9710, #6063, #1921, #7432 ) ) ;
#2512=FACE_OUTER_BOUND ( 'NONE', #7420, .T. ) ;
#2516=EDGE_CURVE ( 'NONE', #1441, #816, #11183, .T. ) ;
#2519=VECTOR ( 'NONE', #11293, 1000.000000000000000 ) ;
#2523=CARTESIAN_POINT ( 'NONE',  ( -6.017756925049793537, 3.000000000000000000, -11.52330688609026232 ) ) ;
#2536=EDGE_LOOP ( 'NONE', ( #10265, #6533, #1609, #3765 ) ) ;
#2538=EDGE_CURVE ( 'NONE', #11094, #10001, #5591, .T. ) ;
#2541=AXIS2_PLACEMENT_3D ( 'NONE', #9215, #7296, #13427 ) ;
#2547=EDGE_CURVE ( 'NONE', #2462, #13403, #13162, .T. ) ;
#2550=ORIENTED_EDGE ( 'NONE', *, *, #1716, .F. ) ;
#2557=EDGE_CURVE ( 'NONE', #3424, #10069, #12758, .T. ) ;
#2559=ORIENTED_EDGE ( 'NONE', *, *, #10713, .F. ) ;
#2562=CARTESIAN_POINT ( 'NONE',  ( -13.86115248177182835, 0.000000000000000000, -5.741477348071267528 ) ) ;
#2563=CARTESIAN_POINT ( 'NONE',  ( 9.375397774054407662, 3.000000000000000000, -11.70905276178460497 ) ) ;
#2572=ORIENTED_EDGE ( 'NONE', *, *, #7675, .F. ) ;
#2578=EDGE_CURVE ( 'NONE', #3210, #5310, #5598, .T. ) ;
#2579=CARTESIAN_POINT ( 'NONE',  ( 9.375397774054407662, 0.000000000000000000, -11.70905276178460497 ) ) ;
#2582=CARTESIAN_POINT ( 'NONE',  ( 2.631756770590782057, 3.000000000000000000, -14.20034848914875347 ) ) ;
#2585=B_SPLINE_SURFACE_WITH_KNOTS ( 'NONE', 3, 1, ( 
 ( #236, #6700 ),
 ( #12840, #2296 ),
 ( #11803, #2366 ),
 ( #4627, #12909 ) ),
 .UNSPECIFIED., .F., .F., .F.,
 ( 4, 4 ),
 ( 2, 2 ),
 ( 0.8181806201944104018, 0.8475986972523573693 ),
 ( 0.000000000000000000, 1.000000000000000000 ),
 .UNSPECIFIED. ) ;
#2591=CARTESIAN_POINT ( 'NONE',  ( -2.264806262022998062, 3.000000000000000000, -14.82803603298499340 ) ) ;
#2596=ORIENTED_EDGE ( 'NONE', *, *, #4648, .T. ) ;
#2602=SURFACE_STYLE_FILL_AREA ( #11988 ) ;
#2624=CARTESIAN_POINT ( 'NONE',  ( -6.025412986832177076, 3.000000000000000000, -13.73660796332610268 ) ) ;
#2628=ORIENTED_EDGE ( 'NONE', *, *, #12319, .T. ) ;
#2630=ADVANCED_FACE ( 'NONE', ( #4766 ), #12004, .F. ) ;
#2631=CARTESIAN_POINT ( 'NONE',  ( -14.39763212228013955, 3.000000000000000000, -1.133238802859595884 ) ) ;
#2633=FACE_OUTER_BOUND ( 'NONE', #5576, .T. ) ;
#2636=CARTESIAN_POINT ( 'NONE',  ( -6.025412986832177076, 3.000000000000000000, -13.73660796332610268 ) ) ;
#2646=ADVANCED_FACE ( 'NONE', ( #5863 ), #3982, .F. ) ;
#2651=B_SPLINE_SURFACE_WITH_KNOTS ( 'NONE', 2, 1, ( 
 ( #8768, #7744 ),
 ( #1048, #2014 ),
 ( #2210, #9311 ) ),
 .UNSPECIFIED., .F., .F., .F.,
 ( 3, 3 ),
 ( 2, 2 ),
 ( 0.000000000000000000, 1.000000000000000000 ),
 ( 0.000000000000000000, 1.000000000000000000 ),
 .UNSPECIFIED. ) ;
#2659=VERTEX_POINT ( 'NONE', #7789 ) ;
#2666=CARTESIAN_POINT ( 'NONE',  ( 9.573149624528804580, 0.000000000000000000, -8.795158114916638681 ) ) ;
#2673=DIRECTION ( 'NONE',  ( -0.000000000000000000, -1.000000000000000000, -0.000000000000000000 ) ) ;
#2674=CARTESIAN_POINT ( 'NONE',  ( 7.499999999999999112, 0.000000000000000000, 0.000000000000000000 ) ) ;
#2677=VERTEX_POINT ( 'NONE', #5711 ) ;
#2685=CARTESIAN_POINT ( 'NONE',  ( -12.30759122141990325, 0.000000000000000000, -6.329356821613475681 ) ) ;
#2687=CARTESIAN_POINT ( 'NONE',  ( -6.025412986832177076, 0.000000000000000000, -13.73660796332610268 ) ) ;
#2689=FACE_OUTER_BOUND ( 'NONE', #5970, .T. ) ;
#2690=VECTOR ( 'NONE', #10705, 1000.000000000000000 ) ;
#2706=CYLINDRICAL_SURFACE ( 'NONE', #3561, 1.500000000000000222 ) ;
#2708=CARTESIAN_POINT ( 'NONE',  ( -1.133238802859761973, 3.000000000000000000, -14.39763212228013067 ) ) ;
#2717=CIRCLE ( 'NONE', #1627, 1.500000000000003997 ) ;
#2722=ADVANCED_FACE ( 'NONE', ( #1593 ), #1915, .F. ) ;
#2732=CARTESIAN_POINT ( 'NONE',  ( 2.830255545554135832, 3.000000000000000000, -12.68816982652952596 ) ) ;
#2740=CARTESIAN_POINT ( 'NONE',  ( 0.5501230721522984979, 0.000000000000000000, -12.98835496148321766 ) ) ;
#2741=APPLICATION_CONTEXT ( 'automotive_design' ) ;
#2742=EDGE_LOOP ( 'NONE', ( #7316, #3855, #5293, #2942 ) ) ;
#2753=ORIENTED_EDGE ( 'NONE', *, *, #10720, .T. ) ;
#2764=( GEOMETRIC_REPRESENTATION_CONTEXT ( 3 ) GLOBAL_UNCERTAINTY_ASSIGNED_CONTEXT ( ( #8059 ) ) GLOBAL_UNIT_ASSIGNED_CONTEXT ( ( #9635, #6539, #2470 ) ) REPRESENTATION_CONTEXT ( 'NONE', 'WORKASPACE' ) );
#2765=CARTESIAN_POINT ( 'NONE',  ( 9.573149624528804580, 0.000000000000000000, -8.795158114916638681 ) ) ;
#2771=EDGE_LOOP ( 'NONE', ( #2209, #11836, #4445, #10124 ) ) ;
#2794=CARTESIAN_POINT ( 'NONE',  ( -14.87484884897975057, 0.000000000000000000, 1.958311002203303453 ) ) ;
#2797=ADVANCED_FACE ( 'NONE', ( #10200 ), #2001, .T. ) ;
#2801=DIRECTION ( 'NONE',  ( 0.000000000000000000, 0.000000000000000000, 1.000000000000000000 ) ) ;
#2805=CARTESIAN_POINT ( 'NONE',  ( 2.264806262022877714, 0.000000000000000000, -14.82803603298501471 ) ) ;
#2807=CARTESIAN_POINT ( 'NONE',  ( -10.25006213149496936, 0.000000000000000000, -9.299128225235415712 ) ) ;
#2814=EDGE_LOOP ( 'NONE', ( #5377, #501, #8859, #385 ) ) ;
#2820=CARTESIAN_POINT ( 'NONE',  ( -5.452638258930639914, 0.000000000000000000, -13.97385902380748313 ) ) ;
#2827=CARTESIAN_POINT ( 'NONE',  ( -6.343077614891082128, 0.000000000000000000, -11.35348748332310720 ) ) ;
#2833=EDGE_LOOP ( 'NONE', ( #9784, #11805, #7652, #9155 ) ) ;
#2838=B_SPLINE_CURVE_WITH_KNOTS ( 'NONE', 3,
 ( #3780, #5992, #9160, #6067 ),
 .UNSPECIFIED., .F., .F.,
 ( 4, 4 ),
 ( 0.000000000000000000, 0.5855695330273008592 ),
 .UNSPECIFIED. ) ;
#2839=ORIENTED_EDGE ( 'NONE', *, *, #12497, .T. ) ;
#2846=CARTESIAN_POINT ( 'NONE',  ( -9.324917476840782982, 0.000000000000000000, -9.065441278446241924 ) ) ;
#2857=FACE_OUTER_BOUND ( 'NONE', #2771, .T. ) ;
#2859=FACE_OUTER_BOUND ( 'NONE', #3174, .T. ) ;
#2863=AXIS2_PLACEMENT_3D ( 'NONE', #6557, #4493, #2419 ) ;
#2870=CARTESIAN_POINT ( 'NONE',  ( 0.1834774187694905023, 3.000000000000000000, -13.00394734430440025 ) ) ;
#2872=ORIENTED_EDGE ( 'NONE', *, *, #12332, .F. ) ;
#2881=CARTESIAN_POINT ( 'NONE',  ( 0.000000000000000000, 3.000000000000000000, 0.000000000000000000 ) ) ;
#2883=CARTESIAN_POINT ( 'NONE',  ( -13.52637830886122572, 0.000000000000000000, -2.928250210355275218 ) ) ;
#2889=EDGE_LOOP ( 'NONE', ( #670, #6294, #3626, #6967 ) ) ;
#2890=CARTESIAN_POINT ( 'NONE',  ( -14.82803603298502360, 3.000000000000000000, -2.264806262022826644 ) ) ;
#2891=VERTEX_POINT ( 'NONE', #13375 ) ;
#2898=B_SPLINE_CURVE_WITH_KNOTS ( 'NONE', 3,
 ( #13071, #1566, #11070, #3553 ),
 .UNSPECIFIED., .F., .F.,
 ( 4, 4 ),
 ( 0.000000000000000000, 0.5855695330273008592 ),
 .UNSPECIFIED. ) ;
#2919=CARTESIAN_POINT ( 'NONE',  ( -12.68816982652953840, 0.000000000000000000, -2.830255545554093644 ) ) ;
#2921=DIRECTION ( 'NONE',  ( 0.000000000000000000, 0.000000000000000000, -1.000000000000000000 ) ) ;
#2922=CARTESIAN_POINT ( 'NONE',  ( -14.82803603298502360, 3.000000000000000000, -2.264806262022826644 ) ) ;
#2935=CARTESIAN_POINT ( 'NONE',  ( -14.87484884897975057, 3.000000000000000000, 1.958311002203303453 ) ) ;
#2937=DIRECTION ( 'NONE',  ( -0.000000000000000000, -1.000000000000000000, -0.000000000000000000 ) ) ;
#2939=EDGE_CURVE ( 'NONE', #6263, #1441, #9356, .T. ) ;
#2942=ORIENTED_EDGE ( 'NONE', *, *, #7785, .T. ) ;
#2945=CARTESIAN_POINT ( 'NONE',  ( -5.452638258930639914, 3.000000000000000000, -13.97385902380748313 ) ) ;
#2946=VECTOR ( 'NONE', #4621, 1000.000000000000000 ) ;
#2952=LINE ( 'NONE', #4954, #9251 ) ;
#2958=CARTESIAN_POINT ( 'NONE',  ( 2.830255545554135832, 0.000000000000000000, -12.68816982652952596 ) ) ;
#2959=CARTESIAN_POINT ( 'NONE',  ( -12.40340517008309185, 0.000000000000000000, -3.893011711613028947 ) ) ;
#2965=CARTESIAN_POINT ( 'NONE',  ( -14.90895795148409420, 3.000000000000000000, 1.650143266773909101 ) ) ;
#2980=EDGE_CURVE ( 'NONE', #117, #5803, #1310, .T. ) ;
#2988=CARTESIAN_POINT ( 'NONE',  ( 10.25006213149504752, 3.000000000000000000, -9.299128225235653744 ) ) ;
#2993=CARTESIAN_POINT ( 'NONE',  ( -8.883544964652065445, 3.000000000000000000, -12.08646469655229438 ) ) ;
#2995=B_SPLINE_CURVE_WITH_KNOTS ( 'NONE', 2,
 ( #6104, #938, #3125 ),
 .UNSPECIFIED., .F., .F.,
 ( 3, 3 ),
 ( 0.000000000000000000, 1.000000000000000000 ),
 .UNSPECIFIED. ) ;
#2998=VERTEX_POINT ( 'NONE', #12548 ) ;
#3002=ORIENTED_EDGE ( 'NONE', *, *, #10108, .F. ) ;
#3007=CARTESIAN_POINT ( 'NONE',  ( -12.08646469655240097, 3.000000000000000000, -8.883544964651921561 ) ) ;
#3008=FACE_BOUND ( 'NONE', #9102, .T. ) ;
#3013=DIRECTION ( 'NONE',  ( -0.000000000000000000, -1.000000000000000000, -0.000000000000000000 ) ) ;
#3033=CARTESIAN_POINT ( 'NONE',  ( -3.542894779577211661, 0.000000000000000000, -12.51336118825813948 ) ) ;
#3060=EDGE_LOOP ( 'NONE', ( #8091, #7329, #1726, #1387 ) ) ;
#3063=CARTESIAN_POINT ( 'NONE',  ( -8.795158114916672432, 0.000000000000000000, -9.573149624528774382 ) ) ;
#3072=CARTESIAN_POINT ( 'NONE',  ( -3.542894779577211661, 0.000000000000000000, -12.51336118825813948 ) ) ;
#3093=CARTESIAN_POINT ( 'NONE',  ( -12.98835496148321944, 3.000000000000000000, -0.5501230721522551992 ) ) ;
#3096=CARTESIAN_POINT ( 'NONE',  ( 9.379342464487701037, 3.000000000000000000, -10.98198414889939301 ) ) ;
#3116=VERTEX_POINT ( 'NONE', #2666 ) ;
#3117=CARTESIAN_POINT ( 'NONE',  ( -10.97318381393799136, 3.000000000000000000, -6.970598036433411693 ) ) ;
#3119=ORIENTED_EDGE ( 'NONE', *, *, #1269, .T. ) ;
#3121=ORIENTED_EDGE ( 'NONE', *, *, #5398, .F. ) ;
#3125=CARTESIAN_POINT ( 'NONE',  ( -12.08646469655240097, 0.000000000000000000, -8.883544964651921561 ) ) ;
#3146=CARTESIAN_POINT ( 'NONE',  ( 8.180229652970799847, 0.000000000000000000, -11.90209577080762848 ) ) ;
#3153=CARTESIAN_POINT ( 'NONE',  ( -8.883544964652065445, 0.000000000000000000, -12.08646469655229438 ) ) ;
#3157=ORIENTED_EDGE ( 'NONE', *, *, #10543, .T. ) ;
#3160=ORIENTED_EDGE ( 'NONE', *, *, #1366, .F. ) ;
#3167=EDGE_CURVE ( 'NONE', #868, #1536, #5731, .T. ) ;
#3169=CARTESIAN_POINT ( 'NONE',  ( 0.6724118135762067183, 0.000000000000000000, -13.82336506795094344 ) ) ;
#3174=EDGE_LOOP ( 'NONE', ( #6209, #10903, #3648, #5215 ) ) ;
#3181=B_SPLINE_CURVE_WITH_KNOTS ( 'NONE', 2,
 ( #11637, #5362, #5167 ),
 .UNSPECIFIED., .F., .F.,
 ( 3, 3 ),
 ( 0.000000000000000000, 1.000000000000000000 ),
 .UNSPECIFIED. ) ;
#3208=DIRECTION ( 'NONE',  ( 0.000000000000000000, 1.000000000000000000, 0.000000000000000000 ) ) ;
#3210=VERTEX_POINT ( 'NONE', #4047 ) ;
#3216=EDGE_CURVE ( 'NONE', #6730, #4765, #2305, .T. ) ;
#3218=CARTESIAN_POINT ( 'NONE',  ( -5.452638258930639914, 0.000000000000000000, -13.97385902380748313 ) ) ;
#3230=CARTESIAN_POINT ( 'NONE',  ( 30.65246752842885058, 0.000000000000000000, -7.988606140548566437 ) ) ;
#3232=CARTESIAN_POINT ( 'NONE',  ( -1.650143266773857142, 3.000000000000000000, -14.90895795148409952 ) ) ;
#3236=ORIENTED_EDGE ( 'NONE', *, *, #12818, .F. ) ;
#3241=ORIENTED_EDGE ( 'NONE', *, *, #7675, .T. ) ;
#3245=CARTESIAN_POINT ( 'NONE',  ( -12.40340517008309185, 3.000000000000000000, -3.893011711613028947 ) ) ;
#3248=FACE_BOUND ( 'NONE', #6666, .T. ) ;
#3253=EDGE_LOOP ( 'NONE', ( #8598, #4261, #2872, #4102 ) ) ;
#3259=CARTESIAN_POINT ( 'NONE',  ( 11.90284147956858085, 3.000000000000000000, -9.133371500908429752 ) ) ;
#3262=ORIENTED_EDGE ( 'NONE', *, *, #4976, .T. ) ;
#3265=DIRECTION ( 'NONE',  ( 0.000000000000000000, 1.000000000000000000, 0.000000000000000000 ) ) ;
#3267=CARTESIAN_POINT ( 'NONE',  ( -12.56843238770841786, 0.000000000000000000, 3.367671042046304741 ) ) ;
#3272=CARTESIAN_POINT ( 'NONE',  ( -13.73660796332618261, 3.000000000000000000, -6.025412986832017204 ) ) ;
#3275=B_SPLINE_CURVE_WITH_KNOTS ( 'NONE', 3,
 ( #13362, #11216, #12197, #3770 ),
 .UNSPECIFIED., .F., .F.,
 ( 4, 4 ),
 ( 0.000000000000000000, 0.5855695330273008592 ),
 .UNSPECIFIED. ) ;
#3276=CARTESIAN_POINT ( 'NONE',  ( 4.227250083625740729, 0.000000000000000000, -13.17831234185050526 ) ) ;
#3292=EDGE_CURVE ( 'NONE', #288, #7860, #3501, .T. ) ;
#3295=CARTESIAN_POINT ( 'NONE',  ( 8.795158114916441505, 0.000000000000000000, -9.573149624528689117 ) ) ;
#3307=CARTESIAN_POINT ( 'NONE',  ( 9.379342464487701037, 3.000000000000000000, -10.98198414889939301 ) ) ;
#3311=CARTESIAN_POINT ( 'NONE',  ( 10.97318381393774089, 3.000000000000000000, -6.970598036433387712 ) ) ;
#3316=ADVANCED_FACE ( 'NONE', ( #8246 ), #11079, .F. ) ;
#3324=VERTEX_POINT ( 'NONE', #6456 ) ;
#3331=CARTESIAN_POINT ( 'NONE',  ( -11.70905276178463872, 0.000000000000000000, -9.375397774054366806 ) ) ;
#3334=ORIENTED_EDGE ( 'NONE', *, *, #3714, .T. ) ;
#3338=ORIENTED_EDGE ( 'NONE', *, *, #7784, .T. ) ;
#3347=DIRECTION ( 'NONE',  ( -0.000000000000000000, -1.000000000000000000, -0.000000000000000000 ) ) ;
#3350=CARTESIAN_POINT ( 'NONE',  ( 3.893011711613070691, 3.000000000000000000, -12.40340517008307231 ) ) ;
#3363=DIRECTION ( 'NONE',  ( 0.000000000000000000, 0.000000000000000000, 1.000000000000000000 ) ) ;
#3367=CIRCLE ( 'NONE', #5570, 1.500000000000000222 ) ;
#3372=ORIENTED_EDGE ( 'NONE', *, *, #12451, .F. ) ;
#3375=CARTESIAN_POINT ( 'NONE',  ( 9.573149624528804580, 3.000000000000000000, -8.795158114916638681 ) ) ;
#3381=DIRECTION ( 'NONE',  ( 0.000000000000000000, 0.000000000000000000, 1.000000000000000000 ) ) ;
#3388=CARTESIAN_POINT ( 'NONE',  ( -14.90895795148411374, 0.000000000000000000, -1.650143266773683726 ) ) ;
#3400=CARTESIAN_POINT ( 'NONE',  ( 6.329356821613516537, 3.000000000000000000, -12.30759122141987305 ) ) ;
#3410=CARTESIAN_POINT ( 'NONE',  ( 3.893011711613070691, 3.000000000000000000, -12.40340517008307231 ) ) ;
#3419=CARTESIAN_POINT ( 'NONE',  ( -7.494008246337227952, 0.000000000000000000, -11.63517940784355886 ) ) ;
#3424=VERTEX_POINT ( 'NONE', #196 ) ;
#3427=CARTESIAN_POINT ( 'NONE',  ( -5.452638258930639914, 0.000000000000000000, -13.97385902380748313 ) ) ;
#3433=CARTESIAN_POINT ( 'NONE',  ( 11.90209577080759296, 0.000000000000000000, -8.180229652970856691 ) ) ;
#3436=ORIENTED_EDGE ( 'NONE', *, *, #888, .F. ) ;
#3437=VERTEX_POINT ( 'NONE', #10522 ) ;
#3442=ORIENTED_EDGE ( 'NONE', *, *, #6934, .F. ) ;
#3445=CARTESIAN_POINT ( 'NONE',  ( -11.52330688609014686, 3.000000000000000000, -6.017756925049552841 ) ) ;
#3449=CARTESIAN_POINT ( 'NONE',  ( 30.80713437936438126, 3.000000000000000000, 0.9994049933487144655 ) ) ;
#3469=ORIENTED_EDGE ( 'NONE', *, *, #6113, .F. ) ;
#3477=CARTESIAN_POINT ( 'NONE',  ( -6.343077614891082128, 3.000000000000000000, -11.35348748332310720 ) ) ;
#3478=B_SPLINE_CURVE_WITH_KNOTS ( 'NONE', 3,
 ( #3602, #7806, #13180, #2919 ),
 .UNSPECIFIED., .F., .F.,
 ( 4, 4 ),
 ( 0.1818127957067485756, 0.2112308727645026418 ),
 .UNSPECIFIED. ) ;
#3479=LINE ( 'NONE', #9500, #730 ) ;
#3483=DIRECTION ( 'NONE',  ( 0.000000000000000000, 0.000000000000000000, -1.000000000000000000 ) ) ;
#3494=CARTESIAN_POINT ( 'NONE',  ( -2.830255545554292151, 3.000000000000000000, -12.68816982652971959 ) ) ;
#3497=CARTESIAN_POINT ( 'NONE',  ( 6.025412986832064277, 3.000000000000000000, -13.73660796332615597 ) ) ;
#3501=CIRCLE ( 'NONE', #13412, 1.499999999999997780 ) ;
#3507=CARTESIAN_POINT ( 'NONE',  ( -14.90895795148411374, 3.000000000000000000, -1.650143266773683726 ) ) ;
#3514=CARTESIAN_POINT ( 'NONE',  ( 2.830255545554135832, 0.000000000000000000, -12.68816982652952596 ) ) ;
#3538=VERTEX_POINT ( 'NONE', #12087 ) ;
#3553=CARTESIAN_POINT ( 'NONE',  ( -12.40340517008309185, 3.000000000000000000, -3.893011711613028947 ) ) ;
#3554=VERTEX_POINT ( 'NONE', #12865 ) ;
#3561=AXIS2_PLACEMENT_3D ( 'NONE', #9114, #7936, #3876 ) ;
#3563=EDGE_CURVE ( 'NONE', #12771, #144, #171, .T. ) ;
#3566=B_SPLINE_SURFACE_WITH_KNOTS ( 'NONE', 3, 1, ( 
 ( #11574, #8514 ),
 ( #10530, #12734 ),
 ( #4329, #3276 ),
 ( #3350, #7631 ) ),
 .UNSPECIFIED., .F., .F., .F.,
 ( 4, 4 ),
 ( 2, 2 ),
 ( 0.000000000000000000, 0.5855695330273008592 ),
 ( 0.000000000000000000, 1.000000000000000000 ),
 .UNSPECIFIED. ) ;
#3567=CARTESIAN_POINT ( 'NONE',  ( -10.98198414889942676, 3.000000000000000000, -9.379342464487661957 ) ) ;
#3570=EDGE_LOOP ( 'NONE', ( #1870, #7741, #6296, #2143 ) ) ;
#3571=AXIS2_PLACEMENT_3D ( 'NONE', #7968, #4947, #11208 ) ;
#3576=VERTEX_POINT ( 'NONE', #4915 ) ;
#3586=CARTESIAN_POINT ( 'NONE',  ( -13.03533457366735426, 0.000000000000000000, -6.217402469309218027 ) ) ;
#3589=CARTESIAN_POINT ( 'NONE',  ( -14.20034848914876235, 0.000000000000000000, -2.631756770590732764 ) ) ;
#3593=ORIENTED_EDGE ( 'NONE', *, *, #10720, .F. ) ;
#3601=CARTESIAN_POINT ( 'NONE',  ( -8.180229652970899323, 0.000000000000000000, -11.90209577080756276 ) ) ;
#3602=CARTESIAN_POINT ( 'NONE',  ( -12.40340517008309185, 0.000000000000000000, -3.893011711613028947 ) ) ;
#3611=EDGE_LOOP ( 'NONE', ( #178, #2274, #10473, #11739 ) ) ;
#3612=EDGE_LOOP ( 'NONE', ( #6342, #8474, #219, #5201 ) ) ;
#3619=FACE_OUTER_BOUND ( 'NONE', #12882, .T. ) ;
#3626=ORIENTED_EDGE ( 'NONE', *, *, #192, .F. ) ;
#3629=EDGE_CURVE ( 'NONE', #3437, #2462, #7237, .T. ) ;
#3632=ORIENTED_EDGE ( 'NONE', *, *, #11103, .F. ) ;
#3639=LINE ( 'NONE', #7838, #1822 ) ;
#3644=ORIENTED_EDGE ( 'NONE', *, *, #4976, .F. ) ;
#3648=ORIENTED_EDGE ( 'NONE', *, *, #10020, .F. ) ;
#3651=CARTESIAN_POINT ( 'NONE',  ( -6.217402469309367241, 3.000000000000000000, -13.03533457366727610 ) ) ;
#3665=CARTESIAN_POINT ( 'NONE',  ( -14.39763212228012534, 3.000000000000000000, 1.133238802859812155 ) ) ;
#3670=CARTESIAN_POINT ( 'NONE',  ( -8.795158114916672432, 0.000000000000000000, -9.573149624528774382 ) ) ;
#3677=ORIENTED_EDGE ( 'NONE', *, *, #1638, .F. ) ;
#3685=CARTESIAN_POINT ( 'NONE',  ( 3.188443874008702661, 3.000000000000000000, -12.60833581801614578 ) ) ;
#3704=CARTESIAN_POINT ( 'NONE',  ( -6.970598036433426792, 3.000000000000000000, -10.97318381393771780 ) ) ;
#3714=EDGE_CURVE ( 'NONE', #12719, #6705, #7130, .T. ) ;
#3716=B_SPLINE_CURVE_WITH_KNOTS ( 'NONE', 2,
 ( #11109, #3796, #7797 ),
 .UNSPECIFIED., .F., .F.,
 ( 3, 3 ),
 ( 0.000000000000000000, 1.000000000000000000 ),
 .UNSPECIFIED. ) ;
#3724=ORIENTED_EDGE ( 'NONE', *, *, #10708, .T. ) ;
#3728=CARTESIAN_POINT ( 'NONE',  ( -13.82336506795094522, 3.000000000000000000, -0.6724118135761603110 ) ) ;
#3729=CARTESIAN_POINT ( 'NONE',  ( 0.000000000000000000, 3.000000000000000000, 0.000000000000000000 ) ) ;
#3730=CARTESIAN_POINT ( 'NONE',  ( 30.66173999750687784, 3.000000000000000000, 0.01003121477750366919 ) ) ;
#3749=AXIS2_PLACEMENT_3D ( 'NONE', #8715, #3347, #7686 ) ;
#3750=B_SPLINE_SURFACE_WITH_KNOTS ( 'NONE', 3, 1, ( 
 ( #10039, #2740 ),
 ( #2870, #4742 ),
 ( #9893, #468 ),
 ( #3902, #8990 ) ),
 .UNSPECIFIED., .F., .F., .F.,
 ( 4, 4 ),
 ( 2, 2 ),
 ( 0.6363612417694253232, 0.6657793188270956231 ),
 ( 0.000000000000000000, 1.000000000000000000 ),
 .UNSPECIFIED. ) ;
#3759=VERTEX_POINT ( 'NONE', #8682 ) ;
#3765=ORIENTED_EDGE ( 'NONE', *, *, #12543, .F. ) ;
#3769=DIRECTION ( 'NONE',  ( -0.000000000000000000, -1.000000000000000000, -0.000000000000000000 ) ) ;
#3770=CARTESIAN_POINT ( 'NONE',  ( 12.08646469655232636, 3.000000000000000000, -8.883544964652022813 ) ) ;
#3774=VERTEX_POINT ( 'NONE', #6350 ) ;
#3780=CARTESIAN_POINT ( 'NONE',  ( -2.264806262022998062, 3.000000000000000000, -14.82803603298499340 ) ) ;
#3782=EDGE_CURVE ( 'NONE', #13024, #5187, #12789, .T. ) ;
#3790=CARTESIAN_POINT ( 'NONE',  ( 8.795158114916441505, 0.000000000000000000, -9.573149624528689117 ) ) ;
#3794=LINE ( 'NONE', #2624, #10670 ) ;
#3796=CARTESIAN_POINT ( 'NONE',  ( -13.86115248177182835, 3.000000000000000000, -5.741477348071267528 ) ) ;
#3803=CIRCLE ( 'NONE', #3571, 1.000000000000000888 ) ;
#3811=CARTESIAN_POINT ( 'NONE',  ( -13.00394681030572208, 0.000000000000000000, -0.1834665838397169235 ) ) ;
#3812=LINE ( 'NONE', #9932, #3960 ) ;
#3825=VERTEX_POINT ( 'NONE', #5515 ) ;
#3829=CARTESIAN_POINT ( 'NONE',  ( 7.494008246337245716, 0.000000000000000000, -11.63517940784380578 ) ) ;
#3831=FACE_BOUND ( 'NONE', #6077, .T. ) ;
#3832=CARTESIAN_POINT ( 'NONE',  ( -2.631756770590896632, 3.000000000000000000, -14.20034848914872505 ) ) ;
#3835=CIRCLE ( 'NONE', #981, 1.500000000000000666 ) ;
#3851=CARTESIAN_POINT ( 'NONE',  ( 3.542895259386137585, 3.000000000000000000, -12.51336047125611017 ) ) ;
#3854=ORIENTED_EDGE ( 'NONE', *, *, #7592, .F. ) ;
#3855=ORIENTED_EDGE ( 'NONE', *, *, #624, .F. ) ;
#3861=CARTESIAN_POINT ( 'NONE',  ( -13.73660796332618261, 0.000000000000000000, -6.025412986832017204 ) ) ;
#3867=EDGE_CURVE ( 'NONE', #3324, #7144, #9718, .T. ) ;
#3873=B_SPLINE_SURFACE_WITH_KNOTS ( 'NONE', 2, 1, ( 
 ( #10856, #2179 ),
 ( #11886, #4446 ),
 ( #7553, #5415 ) ),
 .UNSPECIFIED., .F., .F., .F.,
 ( 3, 3 ),
 ( 2, 2 ),
 ( 0.000000000000000000, 1.000000000000000000 ),
 ( 0.000000000000000000, 1.000000000000000000 ),
 .UNSPECIFIED. ) ;
#3874=ORIENTED_EDGE ( 'NONE', *, *, #224, .T. ) ;
#3876=DIRECTION ( 'NONE',  ( 0.000000000000000000, 0.000000000000000000, -1.000000000000000000 ) ) ;
#3879=CARTESIAN_POINT ( 'NONE',  ( -6.329356821613726147, 3.000000000000000000, -12.30759122142001338 ) ) ;
#3885=EDGE_CURVE ( 'NONE', #12227, #11094, #5394, .T. ) ;
#3887=EDGE_CURVE ( 'NONE', #746, #7144, #10570, .T. ) ;
#3890=CARTESIAN_POINT ( 'NONE',  ( 7.499999999999999112, 3.000000000000000000, 0.000000000000000000 ) ) ;
#3892=CARTESIAN_POINT ( 'NONE',  ( -14.90895795148409420, 0.000000000000000000, 1.650143266773909101 ) ) ;
#3894=DIRECTION ( 'NONE',  ( 0.000000000000000000, -0.000000000000000000, -1.000000000000000000 ) ) ;
#3895=CARTESIAN_POINT ( 'NONE',  ( 9.573149624528804580, 3.000000000000000000, -8.795158114916638681 ) ) ;
#3898=ORIENTED_EDGE ( 'NONE', *, *, #866, .F. ) ;
#3902=CARTESIAN_POINT ( 'NONE',  ( -0.5501230721523990841, 3.000000000000000000, -12.98835496148299384 ) ) ;
#3904=CARTESIAN_POINT ( 'NONE',  ( 7.499999999999999112, 0.000000000000000000, 0.000000000000000000 ) ) ;
#3913=CARTESIAN_POINT ( 'NONE',  ( -10.97318381393799136, 0.000000000000000000, -6.970598036433411693 ) ) ;
#3916=VERTEX_POINT ( 'NONE', #11102 ) ;
#3917=PRODUCT_DEFINITION_CONTEXT ( 'detailed design', #2741, 'design' ) ;
#3922=ORIENTED_EDGE ( 'NONE', *, *, #12261, .T. ) ;
#3926=CARTESIAN_POINT ( 'NONE',  ( -8.795158114916672432, 3.000000000000000000, -9.573149624528774382 ) ) ;
#3944=CARTESIAN_POINT ( 'NONE',  ( -1.133238802859761973, 3.000000000000000000, -14.39763212228013067 ) ) ;
#3945=CARTESIAN_POINT ( 'NONE',  ( 11.63517940784358196, 3.000000000000000000, -7.494008246337187096 ) ) ;
#3948=VERTEX_POINT ( 'NONE', #13028 ) ;
#3958=CARTESIAN_POINT ( 'NONE',  ( -14.82803603298498629, 3.000000000000000000, 2.264806262023049577 ) ) ;
#3960=VECTOR ( 'NONE', #12233, 1000.000000000000000 ) ;
#3962=CARTESIAN_POINT ( 'NONE',  ( -2.830255545554292151, 0.000000000000000000, -12.68816982652971959 ) ) ;
#3966=ORIENTED_EDGE ( 'NONE', *, *, #9788, .T. ) ;
#3973=DIRECTION ( 'NONE',  ( 0.000000000000000000, 1.000000000000000000, 0.000000000000000000 ) ) ;
#3976=ADVANCED_FACE ( 'NONE', ( #7996 ), #10401, .F. ) ;
#3981=CARTESIAN_POINT ( 'NONE',  ( 3.542895259386137585, 0.000000000000000000, -12.51336047125611017 ) ) ;
#3982=B_SPLINE_SURFACE_WITH_KNOTS ( 'NONE', 3, 1, ( 
 ( #3507, #419 ),
 ( #10819, #8804 ),
 ( #7718, #5651 ),
 ( #1388, #9915 ) ),
 .UNSPECIFIED., .F., .F., .F.,
 ( 4, 4 ),
 ( 2, 2 ),
 ( 0.000000000000000000, 0.5855695330273008592 ),
 ( 0.000000000000000000, 1.000000000000000000 ),
 .UNSPECIFIED. ) ;
#3988=DIRECTION ( 'NONE',  ( -0.000000000000000000, -1.000000000000000000, -0.000000000000000000 ) ) ;
#3997=CARTESIAN_POINT ( 'NONE',  ( 1.650143266773734796, 0.000000000000000000, -14.90895795148410841 ) ) ;
#4001=AXIS2_PLACEMENT_3D ( 'NONE', #13216, #12056, #7978 ) ;
#4002=ORIENTED_EDGE ( 'NONE', *, *, #9779, .F. ) ;
#4005=MANIFOLD_SOLID_BREP ( 'Boss-Extrude1', #4212 ) ;
#4007=EDGE_CURVE ( 'NONE', #11354, #12771, #701, .T. ) ;
#4010=CARTESIAN_POINT ( 'NONE',  ( -14.90895795148409420, 0.000000000000000000, 1.650143266773909101 ) ) ;
#4011=CIRCLE ( 'NONE', #6653, 12.99999999999977973 ) ;
#4015=CARTESIAN_POINT ( 'NONE',  ( 11.70905276178455878, 0.000000000000000000, -9.375397774054460953 ) ) ;
#4021=DIRECTION ( 'NONE',  ( -0.000000000000000000, -1.000000000000000000, -0.000000000000000000 ) ) ;
#4029=ORIENTED_EDGE ( 'NONE', *, *, #7416, .F. ) ;
#4038=CARTESIAN_POINT ( 'NONE',  ( -12.30759122141990325, 3.000000000000000000, -6.329356821613475681 ) ) ;
#4042=VERTEX_POINT ( 'NONE', #974 ) ;
#4047=CARTESIAN_POINT ( 'NONE',  ( 0.000000000000000000, 0.000000000000000000, -1.500000000000000222 ) ) ;
#4087=CARTESIAN_POINT ( 'NONE',  ( -0.5501230721523990841, 3.000000000000000000, -12.98835496148299384 ) ) ;
#4097=VERTEX_POINT ( 'NONE', #3230 ) ;
#4100=EDGE_CURVE ( 'NONE', #3538, #9570, #1300, .T. ) ;
#4102=ORIENTED_EDGE ( 'NONE', *, *, #4007, .T. ) ;
#4103=DIRECTION ( 'NONE',  ( 0.000000000000000000, 0.000000000000000000, -1.000000000000000000 ) ) ;
#4104=DIRECTION ( 'NONE',  ( -0.9893737785712105604, -0.000000000000000000, 0.1453943818575021141 ) ) ;
#4110=CARTESIAN_POINT ( 'NONE',  ( 30.79170750349150509, 3.000000000000000000, -0.0004760053210284623249 ) ) ;
#4111=CARTESIAN_POINT ( 'NONE',  ( 30.79170750349150509, 3.000000000000000000, -0.0004760053210284623249 ) ) ;
#4113=LINE ( 'NONE', #629, #1623 ) ;
#4117=CARTESIAN_POINT ( 'NONE',  ( -11.52330688609014686, 0.000000000000000000, -6.017756925049552841 ) ) ;
#4119=CARTESIAN_POINT ( 'NONE',  ( 2.264806262022877714, 0.000000000000000000, -14.82803603298501471 ) ) ;
#4120=CARTESIAN_POINT ( 'NONE',  ( -11.17001009226120445, 3.000000000000000000, -6.660869730750943241 ) ) ;
#4126=ORIENTED_EDGE ( 'NONE', *, *, #2939, .T. ) ;
#4129=CARTESIAN_POINT ( 'NONE',  ( 8.795158114916441505, 3.000000000000000000, -9.573149624528689117 ) ) ;
#4133=CARTESIAN_POINT ( 'NONE',  ( -11.70905276178463872, 3.000000000000000000, -9.375397774054366806 ) ) ;
#4146=CARTESIAN_POINT ( 'NONE',  ( 6.970598036433451661, 3.000000000000000000, -10.97318381393796294 ) ) ;
#4155=CARTESIAN_POINT ( 'NONE',  ( 7.499999999999999112, 0.000000000000000000, 1.499999999999997780 ) ) ;
#4159=EDGE_CURVE ( 'NONE', #2677, #12749, #306, .T. ) ;
#4162=CARTESIAN_POINT ( 'NONE',  ( -2.830255545554292151, 3.000000000000000000, -12.68816982652971959 ) ) ;
#4166=CYLINDRICAL_SURFACE ( 'NONE', #1568, 12.99999999999977973 ) ;
#4182=CARTESIAN_POINT ( 'NONE',  ( -14.82803603298502360, 0.000000000000000000, -2.264806262022826644 ) ) ;
#4183=CYLINDRICAL_SURFACE ( 'NONE', #4258, 1.499999999999997780 ) ;
#4193=CARTESIAN_POINT ( 'NONE',  ( -14.20034848914871795, 0.000000000000000000, 2.631756770590945482 ) ) ;
#4198=CARTESIAN_POINT ( 'NONE',  ( 7.499999999999999112, 3.000000000000000000, 0.000000000000000000 ) ) ;
#4202=EDGE_CURVE ( 'NONE', #6430, #1110, #11670, .T. ) ;
#4210=CARTESIAN_POINT ( 'NONE',  ( -9.133371500908470608, 0.000000000000000000, -11.90284147956855065 ) ) ;
#4212=CLOSED_SHELL ( 'NONE', ( #9843, #12684, #8661, #9142, #12513, #10660, #4820, #2630, #2797, #10505, #700, #3316, #6262, #6772, #1206, #5901, #13575, #7091, #3976, #4624, #8083, #13182, #5086, #8767, #7569, #10700, #12154, #10890, #1221, #5432, #5326, #6181, #10852, #520, #429, #9613, #12923, #9190, #5389, #10924, #5096, #12297, #6506, #11638, #12454, #2722, #11560, #12246, #12495, #7076, #1705, #2646, #567, #2127, #9955, #9755, #1772, #6337, #6740, #12328, #5153, #2039, #8575, #6090 ) ) ;
#4213=FACE_OUTER_BOUND ( 'NONE', #9232, .T. ) ;
#4215=CARTESIAN_POINT ( 'NONE',  ( -12.68816982652970893, 0.000000000000000000, 2.830255545554337004 ) ) ;
#4219=B_SPLINE_SURFACE_WITH_KNOTS ( 'NONE', 2, 1, ( 
 ( #3272, #10669 ),
 ( #7489, #2330 ),
 ( #9685, #8449 ) ),
 .UNSPECIFIED., .F., .F., .F.,
 ( 3, 3 ),
 ( 2, 2 ),
 ( 0.000000000000000000, 1.000000000000000000 ),
 ( 0.000000000000000000, 1.000000000000000000 ),
 .UNSPECIFIED. ) ;
#4224=ORIENTED_EDGE ( 'NONE', *, *, #4509, .F. ) ;
#4229=ORIENTED_EDGE ( 'NONE', *, *, #7893, .T. ) ;
#4254=CARTESIAN_POINT ( 'NONE',  ( 2.928250210355320959, 0.000000000000000000, -13.52637830886121506 ) ) ;
#4258=AXIS2_PLACEMENT_3D ( 'NONE', #10262, #891, #11298 ) ;
#4261=ORIENTED_EDGE ( 'NONE', *, *, #8879, .F. ) ;
#4264=DIRECTION ( 'NONE',  ( -0.000000000000000000, -1.000000000000000000, 0.000000000000000000 ) ) ;
#4268=CARTESIAN_POINT ( 'NONE',  ( 6.025412986832064277, 0.000000000000000000, -13.73660796332615597 ) ) ;
#4285=DIRECTION ( 'NONE',  ( -0.000000000000000000, -1.000000000000000000, -0.000000000000000000 ) ) ;
#4294=CARTESIAN_POINT ( 'NONE',  ( -9.065441275458884007, 3.000000000000000000, -9.324917484779556176 ) ) ;
#4297=VERTEX_POINT ( 'NONE', #10943 ) ;
#4298=B_SPLINE_CURVE_WITH_KNOTS ( 'NONE', 3,
 ( #6368, #4038, #7279, #127 ),
 .UNSPECIFIED., .F., .F.,
 ( 4, 4 ),
 ( 0.000000000000000000, 0.5855695330273008592 ),
 .UNSPECIFIED. ) ;
#4299=ORIENTED_EDGE ( 'NONE', *, *, #5046, .F. ) ;
#4303=CARTESIAN_POINT ( 'NONE',  ( -5.452638258930639914, 3.000000000000000000, -13.97385902380748313 ) ) ;
#4308=B_SPLINE_CURVE_WITH_KNOTS ( 'NONE', 2,
 ( #12716, #3259, #11676 ),
 .UNSPECIFIED., .F., .F.,
 ( 3, 3 ),
 ( 0.000000000000000000, 1.000000000000000000 ),
 .UNSPECIFIED. ) ;
#4324=CARTESIAN_POINT ( 'NONE',  ( 6.970598036433451661, 0.000000000000000000, -10.97318381393796294 ) ) ;
#4325=CARTESIAN_POINT ( 'NONE',  ( 9.573149624528804580, 0.000000000000000000, -8.795158114916638681 ) ) ;
#4328=CARTESIAN_POINT ( 'NONE',  ( 7.499999999999999112, 3.000000000000000000, -1.499999999999997780 ) ) ;
#4329=CARTESIAN_POINT ( 'NONE',  ( 4.227250083625740729, 3.000000000000000000, -13.17831234185050526 ) ) ;
#4330=B_SPLINE_SURFACE_WITH_KNOTS ( 'NONE', 3, 1, ( 
 ( #12026, #511 ),
 ( #9867, #721 ),
 ( #2708, #10975 ),
 ( #5810, #5881 ) ),
 .UNSPECIFIED., .F., .F., .F.,
 ( 4, 4 ),
 ( 2, 2 ),
 ( 0.000000000000000000, 0.5855695330273008592 ),
 ( 0.000000000000000000, 1.000000000000000000 ),
 .UNSPECIFIED. ) ;
#4336=EDGE_CURVE ( 'NONE', #3576, #11340, #9972, .T. ) ;
#4343=CARTESIAN_POINT ( 'NONE',  ( -9.375397774054503586, 0.000000000000000000, -11.70905276178452503 ) ) ;
#4345=CARTESIAN_POINT ( 'NONE',  ( -11.70905276178464050, 3.000000000000000000, -9.375397774054366806 ) ) ;
#4349=ORIENTED_EDGE ( 'NONE', *, *, #13267, .F. ) ;
#4351=CARTESIAN_POINT ( 'NONE',  ( -5.452638258930639914, 3.000000000000000000, -13.97385902380748313 ) ) ;
#4367=CARTESIAN_POINT ( 'NONE',  ( -12.98835496148299207, 0.000000000000000000, 0.5501230721524459355 ) ) ;
#4376=EDGE_CURVE ( 'NONE', #7949, #10891, #11470, .T. ) ;
#4396=ORIENTED_EDGE ( 'NONE', *, *, #8629, .T. ) ;
#4398=EDGE_CURVE ( 'NONE', #3759, #5524, #9284, .T. ) ;
#4401=CARTESIAN_POINT ( 'NONE',  ( 0.000000000000000000, 0.000000000000000000, 0.000000000000000000 ) ) ;
#4402=DIRECTION ( 'NONE',  ( -0.000000000000000000, -1.000000000000000000, 0.000000000000000000 ) ) ;
#4406=CARTESIAN_POINT ( 'NONE',  ( -12.40340517008309185, 3.000000000000000000, -3.893011711613028947 ) ) ;
#4413=CARTESIAN_POINT ( 'NONE',  ( -12.98835496148299207, 0.000000000000000000, 0.5501230721524460465 ) ) ;
#4421=DIRECTION ( 'NONE',  ( 0.000000000000000000, -0.000000000000000000, -1.000000000000000000 ) ) ;
#4427=EDGE_CURVE ( 'NONE', #11094, #5187, #4874, .T. ) ;
#4437=CYLINDRICAL_SURFACE ( 'NONE', #11684, 1.500000000000000222 ) ;
#4443=CARTESIAN_POINT ( 'NONE',  ( 4.227250083625740729, 3.000000000000000000, -13.17831234185050526 ) ) ;
#4445=ORIENTED_EDGE ( 'NONE', *, *, #5021, .T. ) ;
#4446=CARTESIAN_POINT ( 'NONE',  ( -14.87484884897978077, 0.000000000000000000, -1.958311002203079187 ) ) ;
#4454=CYLINDRICAL_SURFACE ( 'NONE', #10661, 1.500000000000000666 ) ;
#4473=B_SPLINE_CURVE_WITH_KNOTS ( 'NONE', 2,
 ( #2313, #6510, #12855 ),
 .UNSPECIFIED., .F., .F.,
 ( 3, 3 ),
 ( 0.000000000000000000, 1.000000000000000000 ),
 .UNSPECIFIED. ) ;
#4476=CARTESIAN_POINT ( 'NONE',  ( 9.133371500908369356, 0.000000000000000000, -11.90284147956862171 ) ) ;
#4477=DIRECTION ( 'NONE',  ( -0.000000000000000000, -1.000000000000000000, -0.000000000000000000 ) ) ;
#4484=ORIENTED_EDGE ( 'NONE', *, *, #4100, .T. ) ;
#4485=CARTESIAN_POINT ( 'NONE',  ( 12.63269908545826503, 3.000000000000000000, -5.340493616518843467 ) ) ;
#4493=DIRECTION ( 'NONE',  ( 0.000000000000000000, 1.000000000000000000, 0.000000000000000000 ) ) ;
#4497=ORIENTED_EDGE ( 'NONE', *, *, #8585, .F. ) ;
#4503=ORIENTED_EDGE ( 'NONE', *, *, #2557, .F. ) ;
#4505=CARTESIAN_POINT ( 'NONE',  ( -14.90895795148409420, 3.000000000000000000, 1.650143266773909101 ) ) ;
#4508=DIRECTION ( 'NONE',  ( -0.000000000000000000, -1.000000000000000000, -0.000000000000000000 ) ) ;
#4509=EDGE_CURVE ( 'NONE', #1456, #868, #8558, .T. ) ;
#4512=CARTESIAN_POINT ( 'NONE',  ( -8.795158114916672432, 3.000000000000000000, -9.573149624528774382 ) ) ;
#4522=B_SPLINE_SURFACE_WITH_KNOTS ( 'NONE', 2, 1, ( 
 ( #8711, #12928 ),
 ( #8506, #3267 ),
 ( #6580, #12726 ) ),
 .UNSPECIFIED., .F., .F., .F.,
 ( 3, 3 ),
 ( 2, 2 ),
 ( 0.000000000000000000, 0.02941149433826504428 ),
 ( 0.000000000000000000, 1.000000000000000000 ),
 .UNSPECIFIED. ) ;
#4525=CARTESIAN_POINT ( 'NONE',  ( 0.5501230721522984979, 3.000000000000000000, -12.98835496148321766 ) ) ;
#4532=VERTEX_POINT ( 'NONE', #4117 ) ;
#4543=CARTESIAN_POINT ( 'NONE',  ( -13.97385902380755240, 3.000000000000000000, -5.452638258930474713 ) ) ;
#4547=ORIENTED_EDGE ( 'NONE', *, *, #8931, .F. ) ;
#4552=ORIENTED_EDGE ( 'NONE', *, *, #11879, .F. ) ;
#4558=CARTESIAN_POINT ( 'NONE',  ( 8.883544964651964193, 3.000000000000000000, -12.08646469655236544 ) ) ;
#4559=B_SPLINE_CURVE_WITH_KNOTS ( 'NONE', 3,
 ( #6574, #8704, #2582, #12920 ),
 .UNSPECIFIED., .F., .F.,
 ( 4, 4 ),
 ( 0.000000000000000000, 0.5855695330273008592 ),
 .UNSPECIFIED. ) ;
#4560=LINE ( 'NONE', #422, #2946 ) ;
#4562=CARTESIAN_POINT ( 'NONE',  ( -14.39763212228012534, 0.000000000000000000, 1.133238802859812155 ) ) ;
#4565=B_SPLINE_SURFACE_WITH_KNOTS ( 'NONE', 3, 1, ( 
 ( #7242, #1941 ),
 ( #6074, #11584 ),
 ( #9434, #3169 ),
 ( #11436, #8391 ) ),
 .UNSPECIFIED., .F., .F., .F.,
 ( 4, 4 ),
 ( 2, 2 ),
 ( 0.000000000000000000, 0.5855695330273008592 ),
 ( 0.000000000000000000, 1.000000000000000000 ),
 .UNSPECIFIED. ) ;
#4567=VERTEX_POINT ( 'NONE', #10666 ) ;
#4575=CARTESIAN_POINT ( 'NONE',  ( -9.573149624528719315, 0.000000000000000000, -8.795158114916407754 ) ) ;
#4577=CARTESIAN_POINT ( 'NONE',  ( 1.836970198721030181E-16, 3.000000000000000000, 1.500000000000000222 ) ) ;
#4581=FACE_OUTER_BOUND ( 'NONE', #11370, .T. ) ;
#4582=EDGE_CURVE ( 'NONE', #8184, #10069, #273, .T. ) ;
#4583=B_SPLINE_CURVE_WITH_KNOTS ( 'NONE', 3,
 ( #7900, #5849, #13152, #8869 ),
 .UNSPECIFIED., .F., .F.,
 ( 4, 4 ),
 ( 0.2727224849193458089, 0.3021405619770169415 ),
 .UNSPECIFIED. ) ;
#4584=B_SPLINE_CURVE_WITH_KNOTS ( 'NONE', 3,
 ( #6105, #13405, #6165, #3063 ),
 .UNSPECIFIED., .F., .F.,
 ( 4, 4 ),
 ( 0.000000000000000000, 0.5855695330273008592 ),
 .UNSPECIFIED. ) ;
#4588=CARTESIAN_POINT ( 'NONE',  ( 6.017756925049591921, 0.000000000000000000, -11.52330688609011844 ) ) ;
#4591=CARTESIAN_POINT ( 'NONE',  ( -11.90209577080766046, 0.000000000000000000, -8.180229652970757215 ) ) ;
#4601=ORIENTED_EDGE ( 'NONE', *, *, #13551, .F. ) ;
#4616=CARTESIAN_POINT ( 'NONE',  ( 30.80713437936438126, 3.000000000000000000, 0.9994049933487144655 ) ) ;
#4618=CARTESIAN_POINT ( 'NONE',  ( -11.52330688609014686, 0.000000000000000000, -6.017756925049552841 ) ) ;
#4620=VECTOR ( 'NONE', #298, 1000.000000000000000 ) ;
#4621=DIRECTION ( 'NONE',  ( -0.000000000000000000, -1.000000000000000000, -0.000000000000000000 ) ) ;
#4624=ADVANCED_FACE ( 'NONE', ( #12729 ), #7438, .F. ) ;
#4627=CARTESIAN_POINT ( 'NONE',  ( 6.017756925049591921, 3.000000000000000000, -11.52330688609011844 ) ) ;
#4636=CARTESIAN_POINT ( 'NONE',  ( -12.08646469655240097, 3.000000000000000000, -8.883544964651921561 ) ) ;
#4638=DIRECTION ( 'NONE',  ( -0.000000000000000000, -1.000000000000000000, -0.000000000000000000 ) ) ;
#4640=CARTESIAN_POINT ( 'NONE',  ( -9.573149624528719315, 3.000000000000000000, -8.795158114916407754 ) ) ;
#4647=ORIENTED_EDGE ( 'NONE', *, *, #12925, .F. ) ;
#4648=EDGE_CURVE ( 'NONE', #6867, #11838, #12104, .T. ) ;
#4649=VECTOR ( 'NONE', #9397, 1000.000000000000000 ) ;
#4656=FACE_OUTER_BOUND ( 'NONE', #11464, .T. ) ;
#4663=ORIENTED_EDGE ( 'NONE', *, *, #11311, .T. ) ;
#4687=CARTESIAN_POINT ( 'NONE',  ( -13.00394572736061605, 3.000000000000000000, 0.1835083749157108701 ) ) ;
#4695=CARTESIAN_POINT ( 'NONE',  ( -3.188443695493920593, 3.000000000000000000, -12.60833606734848189 ) ) ;
#4700=ORIENTED_EDGE ( 'NONE', *, *, #8756, .F. ) ;
#4709=CARTESIAN_POINT ( 'NONE',  ( -14.90895795148409420, 3.000000000000000000, 1.650143266773909101 ) ) ;
#4725=EDGE_CURVE ( 'NONE', #13403, #9256, #52, .T. ) ;
#4726=ORIENTED_EDGE ( 'NONE', *, *, #2547, .T. ) ;
#4727=CARTESIAN_POINT ( 'NONE',  ( 30.73000000000000043, 3.000000000000000000, -5.500000000000003553 ) ) ;
#4742=CARTESIAN_POINT ( 'NONE',  ( 0.1834774187694905023, 0.000000000000000000, -13.00394734430440025 ) ) ;
#4745=B_SPLINE_SURFACE_WITH_KNOTS ( 'NONE', 3, 1, ( 
 ( #801, #8345 ),
 ( #3945, #11530 ),
 ( #8147, #12514 ),
 ( #2095, #12379 ) ),
 .UNSPECIFIED., .F., .F., .F.,
 ( 4, 4 ),
 ( 2, 2 ),
 ( 0.000000000000000000, 0.5855695330273008592 ),
 ( 0.000000000000000000, 1.000000000000000000 ),
 .UNSPECIFIED. ) ;
#4751=CARTESIAN_POINT ( 'NONE',  ( 9.375397774054407662, 0.000000000000000000, -11.70905276178460497 ) ) ;
#4765=VERTEX_POINT ( 'NONE', #9135 ) ;
#4766=FACE_OUTER_BOUND ( 'NONE', #4967, .T. ) ;
#4767=CARTESIAN_POINT ( 'NONE',  ( -8.795158114916672432, 0.000000000000000000, -9.573149624528774382 ) ) ;
#4780=CARTESIAN_POINT ( 'NONE',  ( -7.494008246337227952, 3.000000000000000000, -11.63517940784355886 ) ) ;
#4783=CARTESIAN_POINT ( 'NONE',  ( 5.452638258930520010, 0.000000000000000000, -13.97385902380752754 ) ) ;
#4788=ORIENTED_EDGE ( 'NONE', *, *, #3885, .T. ) ;
#4796=FACE_OUTER_BOUND ( 'NONE', #11403, .T. ) ;
#4806=CARTESIAN_POINT ( 'NONE',  ( 12.48730470360076161, 3.000000000000000000, -6.329867395090054139 ) ) ;
#4812=LINE ( 'NONE', #5912, #717 ) ;
#4820=ADVANCED_FACE ( 'NONE', ( #3831, #3008, #13350, #6107, #13408 ), #7214, .T. ) ;
#4821=ORIENTED_EDGE ( 'NONE', *, *, #8249, .F. ) ;
#4824=DIRECTION ( 'NONE',  ( -0.000000000000000000, -1.000000000000000000, -0.000000000000000000 ) ) ;
#4828=FACE_OUTER_BOUND ( 'NONE', #7514, .T. ) ;
#4831=VERTEX_POINT ( 'NONE', #12320 ) ;
#4840=FACE_OUTER_BOUND ( 'NONE', #2536, .T. ) ;
#4852=ORIENTED_EDGE ( 'NONE', *, *, #12742, .F. ) ;
#4867=ORIENTED_EDGE ( 'NONE', *, *, #9280, .T. ) ;
#4874=LINE ( 'NONE', #7164, #8151 ) ;
#4885=AXIS2_PLACEMENT_3D ( 'NONE', #13253, #12085, #12231 ) ;
#4888=CARTESIAN_POINT ( 'NONE',  ( 3.542895259386137585, 0.000000000000000000, -12.51336047125611017 ) ) ;
#4899=EDGE_CURVE ( 'NONE', #816, #11204, #10162, .T. ) ;
#4914=CARTESIAN_POINT ( 'NONE',  ( -8.883544964652065445, 3.000000000000000000, -12.08646469655229438 ) ) ;
#4915=CARTESIAN_POINT ( 'NONE',  ( -2.830255545554292151, 3.000000000000000000, -12.68816982652971959 ) ) ;
#4947=DIRECTION ( 'NONE',  ( 0.000000000000000000, 1.000000000000000000, -0.000000000000000000 ) ) ;
#4954=CARTESIAN_POINT ( 'NONE',  ( -0.5501230721523990841, 3.000000000000000000, -12.98835496148299384 ) ) ;
#4958=ORIENTED_EDGE ( 'NONE', *, *, #1537, .T. ) ;
#4965=CARTESIAN_POINT ( 'NONE',  ( 9.375397774054407662, 3.000000000000000000, -11.70905276178460497 ) ) ;
#4966=ORIENTED_EDGE ( 'NONE', *, *, #565, .T. ) ;
#4967=EDGE_LOOP ( 'NONE', ( #4663, #7480, #1439, #12659 ) ) ;
#4969=CARTESIAN_POINT ( 'NONE',  ( -13.52637830886139092, 0.000000000000000000, 2.928250210355532790 ) ) ;
#4970=( LENGTH_UNIT ( ) NAMED_UNIT ( * ) SI_UNIT ( .MILLI., .METRE. ) );
#4971=CARTESIAN_POINT ( 'NONE',  ( -9.299128225235689271, 3.000000000000000000, -10.25006213149501555 ) ) ;
#4976=EDGE_CURVE ( 'NONE', #8568, #4097, #1975, .T. ) ;
#4984=CARTESIAN_POINT ( 'NONE',  ( 12.08646469655232636, 3.000000000000000000, -8.883544964652022813 ) ) ;
#5000=DIRECTION ( 'NONE',  ( 0.000000000000000000, 1.000000000000000000, 0.000000000000000000 ) ) ;
#5017=CARTESIAN_POINT ( 'NONE',  ( -14.90895795148411374, 3.000000000000000000, -1.650143266773683726 ) ) ;
#5018=CARTESIAN_POINT ( 'NONE',  ( 2.830255545554135832, 3.000000000000000000, -12.68816982652952596 ) ) ;
#5019=EDGE_CURVE ( 'NONE', #13428, #10501, #4308, .T. ) ;
#5021=EDGE_CURVE ( 'NONE', #12534, #288, #2234, .T. ) ;
#5024=EDGE_LOOP ( 'NONE', ( #1553, #4601, #1533, #12899 ) ) ;
#5037=ORIENTED_EDGE ( 'NONE', *, *, #5308, .F. ) ;
#5039=CARTESIAN_POINT ( 'NONE',  ( 7.499999999999999112, 0.000000000000000000, -1.499999999999997780 ) ) ;
#5043=CARTESIAN_POINT ( 'NONE',  ( -11.90209577080766046, 0.000000000000000000, -8.180229652970757215 ) ) ;
#5044=CARTESIAN_POINT ( 'NONE',  ( 2.264806262022877714, 3.000000000000000000, -14.82803603298501471 ) ) ;
#5046=EDGE_CURVE ( 'NONE', #1608, #10985, #4473, .T. ) ;
#5049=CARTESIAN_POINT ( 'NONE',  ( -14.90895795148411374, 0.000000000000000000, -1.650143266773683726 ) ) ;
#5050=CARTESIAN_POINT ( 'NONE',  ( -0.5501230721523990841, 3.000000000000000000, -12.98835496148299384 ) ) ;
#5076=CARTESIAN_POINT ( 'NONE',  ( -3.893011711613112880, 3.000000000000000000, -12.40340517008282717 ) ) ;
#5084=CARTESIAN_POINT ( 'NONE',  ( 10.98198414889934682, 0.000000000000000000, -9.379342464487748998 ) ) ;
#5086=ADVANCED_FACE ( 'NONE', ( #10846 ), #82, .F. ) ;
#5092=EDGE_LOOP ( 'NONE', ( #1908, #7529, #8317, #580 ) ) ;
#5095=AXIS2_PLACEMENT_3D ( 'NONE', #2158, #4021, #926 ) ;
#5096=ADVANCED_FACE ( 'NONE', ( #8627 ), #8412, .F. ) ;
#5109=CARTESIAN_POINT ( 'NONE',  ( 0.000000000000000000, 3.000000000000000000, 0.000000000000000000 ) ) ;
#5125=ORIENTED_EDGE ( 'NONE', *, *, #7422, .T. ) ;
#5130=B_SPLINE_CURVE_WITH_KNOTS ( 'NONE', 3,
 ( #9884, #5833, #395, #5895 ),
 .UNSPECIFIED., .F., .F.,
 ( 4, 4 ),
 ( 0.000000000000000000, 0.5855695330273008592 ),
 .UNSPECIFIED. ) ;
#5135=SHAPE_REPRESENTATION ( 'gear-link-2', ( #10007 ), #6949 ) ;
#5138=DIRECTION ( 'NONE',  ( -0.000000000000000000, -1.000000000000000000, -0.000000000000000000 ) ) ;
#5151=EDGE_LOOP ( 'NONE', ( #7966, #13171, #269, #6371 ) ) ;
#5153=ADVANCED_FACE ( 'NONE', ( #2512 ), #4437, .F. ) ;
#5159=CARTESIAN_POINT ( 'NONE',  ( -12.98835496148321944, 3.000000000000000000, -0.5501230721522551992 ) ) ;
#5167=CARTESIAN_POINT ( 'NONE',  ( -2.264806262022998062, 0.000000000000000000, -14.82803603298499340 ) ) ;
#5171=EDGE_CURVE ( 'NONE', #12311, #11204, #2173, .T. ) ;
#5172=AXIS2_PLACEMENT_3D ( 'NONE', #9445, #28, #5445 ) ;
#5173=B_SPLINE_CURVE_WITH_KNOTS ( 'NONE', 3,
 ( #12025, #11042, #3665, #4709 ),
 .UNSPECIFIED., .F., .F.,
 ( 4, 4 ),
 ( 0.000000000000000000, 0.5855695330273008592 ),
 .UNSPECIFIED. ) ;
#5179=CARTESIAN_POINT ( 'NONE',  ( -13.17831234185052836, 0.000000000000000000, -4.227250083625696320 ) ) ;
#5187=VERTEX_POINT ( 'NONE', #11187 ) ;
#5188=CARTESIAN_POINT ( 'NONE',  ( -3.893011711613112880, 3.000000000000000000, -12.40340517008282717 ) ) ;
#5198=LINE ( 'NONE', #9328, #6050 ) ;
#5199=ORIENTED_EDGE ( 'NONE', *, *, #1970, .T. ) ;
#5201=ORIENTED_EDGE ( 'NONE', *, *, #12054, .T. ) ;
#5202=EDGE_CURVE ( 'NONE', #12679, #2677, #376, .T. ) ;
#5208=CARTESIAN_POINT ( 'NONE',  ( 6.329356821613516537, 0.000000000000000000, -12.30759122141987305 ) ) ;
#5215=ORIENTED_EDGE ( 'NONE', *, *, #11732, .T. ) ;
#5221=CARTESIAN_POINT ( 'NONE',  ( -8.883544964652065445, 3.000000000000000000, -12.08646469655229438 ) ) ;
#5225=VERTEX_POINT ( 'NONE', #2922 ) ;
#5227=LINE ( 'NONE', #10327, #11498 ) ;
#5232=EDGE_CURVE ( 'NONE', #9256, #1608, #12866, .T. ) ;
#5247=VERTEX_POINT ( 'NONE', #5948 ) ;
#5249=LINE ( 'NONE', #4146, #5613 ) ;
#5258=EDGE_LOOP ( 'NONE', ( #1748, #13382, #1795, #5989 ) ) ;
#5268=CARTESIAN_POINT ( 'NONE',  ( -6.970598036433426792, 0.000000000000000000, -10.97318381393771780 ) ) ;
#5273=CARTESIAN_POINT ( 'NONE',  ( -12.98835496148299207, 0.000000000000000000, 0.5501230721524459355 ) ) ;
#5275=ORIENTED_EDGE ( 'NONE', *, *, #12451, .T. ) ;
#5284=CARTESIAN_POINT ( 'NONE',  ( -11.35348746973813761, 0.000000000000000000, -6.343077501554963860 ) ) ;
#5288=STYLED_ITEM('',(#13663),#4005);
#5293=ORIENTED_EDGE ( 'NONE', *, *, #3629, .F. ) ;
#5296=CARTESIAN_POINT ( 'NONE',  ( 6.217402469309262436, 0.000000000000000000, -13.03533457366732939 ) ) ;
#5305=ORIENTED_EDGE ( 'NONE', *, *, #2516, .T. ) ;
#5307=VECTOR ( 'NONE', #8546, 1000.000000000000000 ) ;
#5308=EDGE_CURVE ( 'NONE', #7949, #6730, #5883, .T. ) ;
#5310=VERTEX_POINT ( 'NONE', #11258 ) ;
#5323=B_SPLINE_SURFACE_WITH_KNOTS ( 'NONE', 3, 1, ( 
 ( #10467, #2959 ),
 ( #827, #11367 ),
 ( #11426, #1929 ),
 ( #6124, #12604 ) ),
 .UNSPECIFIED., .F., .F., .F.,
 ( 4, 4 ),
 ( 2, 2 ),
 ( 0.1818127957067485756, 0.2112308727645026418 ),
 ( 0.000000000000000000, 1.000000000000000000 ),
 .UNSPECIFIED. ) ;
#5326=ADVANCED_FACE ( 'NONE', ( #6543 ), #10932, .F. ) ;
#5328=EDGE_LOOP ( 'NONE', ( #7337, #13110, #11975, #12262 ) ) ;
#5335=LINE ( 'NONE', #3007, #953 ) ;
#5336=DIRECTION ( 'NONE',  ( -0.000000000000000000, -1.000000000000000000, -0.000000000000000000 ) ) ;
#5337=FACE_OUTER_BOUND ( 'NONE', #6103, .T. ) ;
#5348=FACE_OUTER_BOUND ( 'NONE', #5761, .T. ) ;
#5354=DIRECTION ( 'NONE',  ( 0.000000000000000000, 1.000000000000000000, 0.000000000000000000 ) ) ;
#5355=DIRECTION ( 'NONE',  ( 0.000000000000000000, 0.000000000000000000, -1.000000000000000000 ) ) ;
#5356=AXIS2_PLACEMENT_3D ( 'NONE', #3890, #9337, #4103 ) ;
#5362=CARTESIAN_POINT ( 'NONE',  ( -1.958311002203252160, 0.000000000000000000, -14.87484884897975768 ) ) ;
#5372=CARTESIAN_POINT ( 'NONE',  ( -9.573149624528719315, 3.000000000000000000, -8.795158114916407754 ) ) ;
#5374=VERTEX_POINT ( 'NONE', #12452 ) ;
#5377=ORIENTED_EDGE ( 'NONE', *, *, #2557, .T. ) ;
#5381=FACE_OUTER_BOUND ( 'NONE', #5393, .T. ) ;
#5386=CARTESIAN_POINT ( 'NONE',  ( 6.970598036433451661, 3.000000000000000000, -10.97318381393796294 ) ) ;
#5389=ADVANCED_FACE ( 'NONE', ( #5434 ), #9934, .F. ) ;
#5393=EDGE_LOOP ( 'NONE', ( #10656, #3593, #3160, #7988 ) ) ;
#5394=B_SPLINE_CURVE_WITH_KNOTS ( 'NONE', 2,
 ( #2359, #8481, #5448 ),
 .UNSPECIFIED., .F., .F.,
 ( 3, 3 ),
 ( 0.000000000000000000, 1.000000000000000000 ),
 .UNSPECIFIED. ) ;
#5398=EDGE_CURVE ( 'NONE', #4831, #3424, #6376, .T. ) ;
#5415=CARTESIAN_POINT ( 'NONE',  ( -14.90895795148411374, 0.000000000000000000, -1.650143266773683726 ) ) ;
#5426=FACE_OUTER_BOUND ( 'NONE', #9048, .T. ) ;
#5428=DIRECTION ( 'NONE',  ( 0.000000000000000000, 0.000000000000000000, -1.000000000000000000 ) ) ;
#5432=ADVANCED_FACE ( 'NONE', ( #7866 ), #4330, .F. ) ;
#5434=FACE_OUTER_BOUND ( 'NONE', #8056, .T. ) ;
#5445=DIRECTION ( 'NONE',  ( 0.000000000000000000, 0.000000000000000000, 1.000000000000000000 ) ) ;
#5448=CARTESIAN_POINT ( 'NONE',  ( -9.375397774054503586, 3.000000000000000000, -11.70905276178452503 ) ) ;
#5461=CARTESIAN_POINT ( 'NONE',  ( 6.017756925049591921, 0.000000000000000000, -11.52330688609011844 ) ) ;
#5462=LINE ( 'NONE', #10912, #12418 ) ;
#5465=B_SPLINE_CURVE_WITH_KNOTS ( 'NONE', 2,
 ( #10080, #7056, #513 ),
 .UNSPECIFIED., .F., .F.,
 ( 3, 3 ),
 ( 0.000000000000000000, 1.000000000000000000 ),
 .UNSPECIFIED. ) ;
#5471=EDGE_CURVE ( 'NONE', #4097, #4297, #8969, .T. ) ;
#5475=EDGE_CURVE ( 'NONE', #13401, #7860, #3812, .T. ) ;
#5484=ORIENTED_EDGE ( 'NONE', *, *, #1716, .T. ) ;
#5486=CARTESIAN_POINT ( 'NONE',  ( 30.73000000000000043, 3.000000000000000000, -2.499999999999995115 ) ) ;
#5494=DIRECTION ( 'NONE',  ( -0.000000000000000000, -1.000000000000000000, -0.000000000000000000 ) ) ;
#5495=B_SPLINE_CURVE_WITH_KNOTS ( 'NONE', 3,
 ( #12445, #5043, #6285, #2020 ),
 .UNSPECIFIED., .F., .F.,
 ( 4, 4 ),
 ( 0.000000000000000000, 0.5855695330273008592 ),
 .UNSPECIFIED. ) ;
#5499=CARTESIAN_POINT ( 'NONE',  ( 5.741477348071313713, 3.000000000000000000, -13.86115248177180703 ) ) ;
#5500=VERTEX_POINT ( 'NONE', #11184 ) ;
#5504=VERTEX_POINT ( 'NONE', #4636 ) ;
#5506=EDGE_CURVE ( 'NONE', #1651, #6481, #3478, .T. ) ;
#5507=ORIENTED_EDGE ( 'NONE', *, *, #935, .F. ) ;
#5514=CARTESIAN_POINT ( 'NONE',  ( -12.68816982652953840, 3.000000000000000000, -2.830255545554093644 ) ) ;
#5515=CARTESIAN_POINT ( 'NONE',  ( -12.40347894490204972, 3.000000000000000000, 3.892776652129660064 ) ) ;
#5524=VERTEX_POINT ( 'NONE', #12568 ) ;
#5540=CARTESIAN_POINT ( 'NONE',  ( 5.452638258930520010, 3.000000000000000000, -13.97385902380752754 ) ) ;
#5548=VECTOR ( 'NONE', #2288, 1000.000000000000000 ) ;
#5550=CARTESIAN_POINT ( 'NONE',  ( 0.1834774187694905023, 3.000000000000000000, -13.00394734430440025 ) ) ;
#5552=B_SPLINE_CURVE_WITH_KNOTS ( 'NONE', 2,
 ( #9305, #2078, #11377 ),
 .UNSPECIFIED., .F., .F.,
 ( 3, 3 ),
 ( 0.000000000000000000, 0.02941149433826504428 ),
 .UNSPECIFIED. ) ;
#5556=CARTESIAN_POINT ( 'NONE',  ( -8.180229652970899323, 0.000000000000000000, -11.90209577080756276 ) ) ;
#5569=CIRCLE ( 'NONE', #13502, 1.000000000000000888 ) ;
#5570=AXIS2_PLACEMENT_3D ( 'NONE', #815, #12471, #2801 ) ;
#5576=EDGE_LOOP ( 'NONE', ( #9909, #11467, #7729, #9598 ) ) ;
#5588=CARTESIAN_POINT ( 'NONE',  ( 2.631756770590782057, 0.000000000000000000, -14.20034848914875347 ) ) ;
#5591=B_SPLINE_CURVE_WITH_KNOTS ( 'NONE', 3,
 ( #10557, #8540, #11525, #6282 ),
 .UNSPECIFIED., .F., .F.,
 ( 4, 4 ),
 ( 0.000000000000000000, 0.5855695330273008592 ),
 .UNSPECIFIED. ) ;
#5594=EDGE_LOOP ( 'NONE', ( #9371, #13542, #11744, #12224 ) ) ;
#5598=CIRCLE ( 'NONE', #5172, 1.500000000000000222 ) ;
#5608=CARTESIAN_POINT ( 'NONE',  ( -9.065441275458884007, 3.000000000000000000, -9.324917484779556176 ) ) ;
#5613=VECTOR ( 'NONE', #6489, 1000.000000000000000 ) ;
#5614=AXIS2_PLACEMENT_3D ( 'NONE', #6879, #5985, #7778 ) ;
#5617=ORIENTED_EDGE ( 'NONE', *, *, #6158, .T. ) ;
#5624=CARTESIAN_POINT ( 'NONE',  ( -12.08646469655240097, 3.000000000000000000, -8.883544964651921561 ) ) ;
#5625=DIRECTION ( 'NONE',  ( 0.000000000000000000, 0.000000000000000000, 1.000000000000000000 ) ) ;
#5626=DIRECTION ( 'NONE',  ( -0.000000000000000000, -1.000000000000000000, -0.000000000000000000 ) ) ;
#5630=ORIENTED_EDGE ( 'NONE', *, *, #6934, .T. ) ;
#5640=B_SPLINE_CURVE_WITH_KNOTS ( 'NONE', 3,
 ( #5076, #8169, #12401, #2945 ),
 .UNSPECIFIED., .F., .F.,
 ( 4, 4 ),
 ( 0.000000000000000000, 0.5855695330273008592 ),
 .UNSPECIFIED. ) ;
#5641=LINE ( 'NONE', #281, #7600 ) ;
#5643=CYLINDRICAL_SURFACE ( 'NONE', #11956, 1.500000000000000666 ) ;
#5644=ORIENTED_EDGE ( 'NONE', *, *, #224, .F. ) ;
#5645=ORIENTED_EDGE ( 'NONE', *, *, #1638, .T. ) ;
#5646=DIRECTION ( 'NONE',  ( -0.000000000000000000, -1.000000000000000000, -0.000000000000000000 ) ) ;
#5651=CARTESIAN_POINT ( 'NONE',  ( -13.82336506795094522, 0.000000000000000000, -0.6724118135761603110 ) ) ;
#5655=DIRECTION ( 'NONE',  ( -0.000000000000000000, -1.000000000000000000, -0.000000000000000000 ) ) ;
#5656=EDGE_CURVE ( 'NONE', #11262, #12351, #12215, .T. ) ;
#5657=CARTESIAN_POINT ( 'NONE',  ( -12.68816982652953840, 0.000000000000000000, -2.830255545554093644 ) ) ;
#5659=ORIENTED_EDGE ( 'NONE', *, *, #9280, .F. ) ;
#5661=B_SPLINE_SURFACE_WITH_KNOTS ( 'NONE', 3, 1, ( 
 ( #6652, #11132 ),
 ( #3477, #9818 ),
 ( #10026, #8979 ),
 ( #13193, #1702 ) ),
 .UNSPECIFIED., .F., .F., .F.,
 ( 4, 4 ),
 ( 2, 2 ),
 ( 0.4545418633443863987, 0.4839599404020549223 ),
 ( 0.000000000000000000, 1.000000000000000000 ),
 .UNSPECIFIED. ) ;
#5662=ORIENTED_EDGE ( 'NONE', *, *, #12086, .F. ) ;
#5667=DIRECTION ( 'NONE',  ( 0.000000000000000000, 0.000000000000000000, 1.000000000000000000 ) ) ;
#5672=CARTESIAN_POINT ( 'NONE',  ( 30.73000000000000043, 3.000000000000000000, -5.500000000000003553 ) ) ;
#5688=ORIENTED_EDGE ( 'NONE', *, *, #5019, .F. ) ;
#5692=CARTESIAN_POINT ( 'NONE',  ( 11.70905276178455878, 3.000000000000000000, -9.375397774054460953 ) ) ;
#5703=FACE_OUTER_BOUND ( 'NONE', #2498, .T. ) ;
#5711=CARTESIAN_POINT ( 'NONE',  ( 5.452638258930520010, 0.000000000000000000, -13.97385902380752754 ) ) ;
#5712=DIRECTION ( 'NONE',  ( 1.000000000000000000, 0.000000000000000000, 0.000000000000000000 ) ) ;
#5714=CARTESIAN_POINT ( 'NONE',  ( -14.39763212228013955, 0.000000000000000000, -1.133238802859595884 ) ) ;
#5715=AXIS2_PLACEMENT_3D ( 'NONE', #6333, #213, #1100 ) ;
#5722=ORIENTED_EDGE ( 'NONE', *, *, #10382, .T. ) ;
#5726=B_SPLINE_SURFACE_WITH_KNOTS ( 'NONE', 3, 1, ( 
 ( #8799, #8740 ),
 ( #483, #1517 ),
 ( #4687, #2352 ),
 ( #12955, #4413 ) ),
 .UNSPECIFIED., .F., .F., .F.,
 ( 4, 4 ),
 ( 2, 2 ),
 ( 0.09090310649439187207, 0.1203211835519651524 ),
 ( 0.000000000000000000, 1.000000000000000000 ),
 .UNSPECIFIED. ) ;
#5731=B_SPLINE_CURVE_WITH_KNOTS ( 'NONE', 2,
 ( #3427, #7639, #11843 ),
 .UNSPECIFIED., .F., .F.,
 ( 3, 3 ),
 ( 0.000000000000000000, 1.000000000000000000 ),
 .UNSPECIFIED. ) ;
#5755=AXIS2_PLACEMENT_3D ( 'NONE', #2237, #2174, #13294 ) ;
#5761=EDGE_LOOP ( 'NONE', ( #166, #1436, #7828, #3334 ) ) ;
#5779=AXIS2_PLACEMENT_3D ( 'NONE', #8773, #7819, #12993 ) ;
#5803=VERTEX_POINT ( 'NONE', #618 ) ;
#5806=EDGE_CURVE ( 'NONE', #11316, #6828, #8997, .T. ) ;
#5807=CARTESIAN_POINT ( 'NONE',  ( -6.970598036433426792, 0.000000000000000000, -10.97318381393771780 ) ) ;
#5810=CARTESIAN_POINT ( 'NONE',  ( -1.650143266773857142, 3.000000000000000000, -14.90895795148409952 ) ) ;
#5820=EDGE_CURVE ( 'NONE', #3324, #13428, #3275, .T. ) ;
#5832=EDGE_CURVE ( 'NONE', #9256, #9763, #2952, .T. ) ;
#5833=CARTESIAN_POINT ( 'NONE',  ( -7.494008246337227952, 3.000000000000000000, -11.63517940784355886 ) ) ;
#5837=CARTESIAN_POINT ( 'NONE',  ( -12.98835496148299207, 3.000000000000000000, 0.5501230721524459355 ) ) ;
#5838=ORIENTED_EDGE ( 'NONE', *, *, #9435, .T. ) ;
#5849=CARTESIAN_POINT ( 'NONE',  ( -11.17001009226120445, 0.000000000000000000, -6.660869730750943241 ) ) ;
#5855=ORIENTED_EDGE ( 'NONE', *, *, #11388, .T. ) ;
#5863=FACE_OUTER_BOUND ( 'NONE', #10171, .T. ) ;
#5881=CARTESIAN_POINT ( 'NONE',  ( -1.650143266773857142, 0.000000000000000000, -14.90895795148409952 ) ) ;
#5883=LINE ( 'NONE', #8017, #12774 ) ;
#5884=DIRECTION ( 'NONE',  ( -0.000000000000000000, -1.000000000000000000, -0.000000000000000000 ) ) ;
#5895=CARTESIAN_POINT ( 'NONE',  ( -8.883544964652065445, 3.000000000000000000, -12.08646469655229438 ) ) ;
#5901=ADVANCED_FACE ( 'NONE', ( #9072 ), #162, .F. ) ;
#5912=CARTESIAN_POINT ( 'NONE',  ( 6.017756925049591921, 3.000000000000000000, -11.52330688609011844 ) ) ;
#5920=ORIENTED_EDGE ( 'NONE', *, *, #12852, .F. ) ;
#5924=DIRECTION ( 'NONE',  ( -0.000000000000000000, -1.000000000000000000, -0.000000000000000000 ) ) ;
#5931=DIRECTION ( 'NONE',  ( -0.000000000000000000, -1.000000000000000000, -0.000000000000000000 ) ) ;
#5932=ORIENTED_EDGE ( 'NONE', *, *, #5021, .F. ) ;
#5944=DIRECTION ( 'NONE',  ( 0.9893737785712105604, -0.000000000000000000, -0.1453943818575020863 ) ) ;
#5948=CARTESIAN_POINT ( 'NONE',  ( 1.650143266773734796, 0.000000000000000000, -14.90895795148410841 ) ) ;
#5951=CARTESIAN_POINT ( 'NONE',  ( 30.79786191028635400, 3.000000000000000000, -6.999232361977355765 ) ) ;
#5955=ORIENTED_EDGE ( 'NONE', *, *, #11879, .T. ) ;
#5963=CARTESIAN_POINT ( 'NONE',  ( 30.80713437936438126, 0.000000000000000000, 0.9994049933487144655 ) ) ;
#5970=EDGE_LOOP ( 'NONE', ( #11369, #10690, #2113, #1376 ) ) ;
#5977=VECTOR ( 'NONE', #7923, 1000.000000000000000 ) ;
#5980=DIRECTION ( 'NONE',  ( -0.000000000000000000, -1.000000000000000000, -0.000000000000000000 ) ) ;
#5982=DIRECTION ( 'NONE',  ( -0.000000000000000000, -1.000000000000000000, 0.000000000000000000 ) ) ;
#5984=FACE_OUTER_BOUND ( 'NONE', #1648, .T. ) ;
#5985=DIRECTION ( 'NONE',  ( -0.1453943818575021141, 0.000000000000000000, -0.9893737785712106714 ) ) ;
#5986=ORIENTED_EDGE ( 'NONE', *, *, #9435, .F. ) ;
#5989=ORIENTED_EDGE ( 'NONE', *, *, #7018, .T. ) ;
#5992=CARTESIAN_POINT ( 'NONE',  ( -2.631756770590896632, 3.000000000000000000, -14.20034848914872505 ) ) ;
#5995=CARTESIAN_POINT ( 'NONE',  ( -7.500000000000000000, 3.000000000000000000, 0.000000000000000000 ) ) ;
#5999=CARTESIAN_POINT ( 'NONE',  ( -6.660869762029062890, 0.000000000000000000, -11.17001010193236610 ) ) ;
#6036=ORIENTED_EDGE ( 'NONE', *, *, #9169, .F. ) ;
#6050=VECTOR ( 'NONE', #12901, 1000.000000000000000 ) ;
#6063=ORIENTED_EDGE ( 'NONE', *, *, #1575, .T. ) ;
#6067=CARTESIAN_POINT ( 'NONE',  ( -2.830255545554292151, 3.000000000000000000, -12.68816982652971959 ) ) ;
#6074=CARTESIAN_POINT ( 'NONE',  ( 1.133238802859644956, 3.000000000000000000, -14.39763212228013600 ) ) ;
#6077=EDGE_LOOP ( 'NONE', ( #502, #132 ) ) ;
#6083=B_SPLINE_SURFACE_WITH_KNOTS ( 'NONE', 3, 1, ( 
 ( #8492, #4367 ),
 ( #1069, #2306 ),
 ( #9733, #12714 ),
 ( #4505, #2167 ) ),
 .UNSPECIFIED., .F., .F., .F.,
 ( 4, 4 ),
 ( 2, 2 ),
 ( 0.000000000000000000, 0.5855695330273008592 ),
 ( 0.000000000000000000, 1.000000000000000000 ),
 .UNSPECIFIED. ) ;
#6090=ADVANCED_FACE ( 'NONE', ( #4656 ), #12868, .F. ) ;
#6100=ORIENTED_EDGE ( 'NONE', *, *, #3292, .F. ) ;
#6103=EDGE_LOOP ( 'NONE', ( #10673, #6744, #13545, #13000 ) ) ;
#6104=CARTESIAN_POINT ( 'NONE',  ( -11.70905276178463872, 0.000000000000000000, -9.375397774054366806 ) ) ;
#6105=CARTESIAN_POINT ( 'NONE',  ( -9.375397774054503586, 0.000000000000000000, -11.70905276178452503 ) ) ;
#6107=FACE_BOUND ( 'NONE', #6407, .T. ) ;
#6109=CARTESIAN_POINT ( 'NONE',  ( -14.20034848914871795, 3.000000000000000000, 2.631756770590945482 ) ) ;
#6113=EDGE_CURVE ( 'NONE', #5504, #3759, #2325, .T. ) ;
#6119=CARTESIAN_POINT ( 'NONE',  ( -9.573149624528719315, 0.000000000000000000, -8.795158114916407754 ) ) ;
#6124=CARTESIAN_POINT ( 'NONE',  ( -12.68816982652953840, 3.000000000000000000, -2.830255545554093644 ) ) ;
#6127=EDGE_LOOP ( 'NONE', ( #11793, #10931, #2572, #10191 ) ) ;
#6133=B_SPLINE_CURVE_WITH_KNOTS ( 'NONE', 3,
 ( #7940, #1619, #2846, #12162 ),
 .UNSPECIFIED., .F., .F.,
 ( 4, 4 ),
 ( 0.3636321741318673806, 0.3930502511895355711 ),
 .UNSPECIFIED. ) ;
#6134=CARTESIAN_POINT ( 'NONE',  ( 9.299128225235451239, 0.000000000000000000, -10.25006213149493561 ) ) ;
#6140=ORIENTED_EDGE ( 'NONE', *, *, #2217, .T. ) ;
#6142=ORIENTED_EDGE ( 'NONE', *, *, #192, .T. ) ;
#6158=EDGE_CURVE ( 'NONE', #12983, #3916, #10541, .T. ) ;
#6165=CARTESIAN_POINT ( 'NONE',  ( -9.299128225235689271, 0.000000000000000000, -10.25006213149501555 ) ) ;
#6174=ORIENTED_EDGE ( 'NONE', *, *, #9373, .T. ) ;
#6181=ADVANCED_FACE ( 'NONE', ( #11201 ), #7282, .F. ) ;
#6182=CARTESIAN_POINT ( 'NONE',  ( -10.97318381393799136, 3.000000000000000000, -6.970598036433411693 ) ) ;
#6186=DIRECTION ( 'NONE',  ( 0.000000000000000000, 0.000000000000000000, -1.000000000000000000 ) ) ;
#6190=CARTESIAN_POINT ( 'NONE',  ( -2.830255545554292151, 0.000000000000000000, -12.68816982652971959 ) ) ;
#6192=ORIENTED_EDGE ( 'NONE', *, *, #6232, .F. ) ;
#6201=LINE ( 'NONE', #7380, #9976 ) ;
#6206=CARTESIAN_POINT ( 'NONE',  ( -11.52330688609014686, 3.000000000000000000, -6.017756925049552841 ) ) ;
#6209=ORIENTED_EDGE ( 'NONE', *, *, #12925, .T. ) ;
#6215=CARTESIAN_POINT ( 'NONE',  ( 8.795158114916441505, 3.000000000000000000, -9.573149624528689117 ) ) ;
#6219=CARTESIAN_POINT ( 'NONE',  ( -12.68816982652970893, 3.000000000000000000, 2.830255545554337004 ) ) ;
#6223=DIRECTION ( 'NONE',  ( -0.000000000000000000, -1.000000000000000000, -0.000000000000000000 ) ) ;
#6229=CIRCLE ( 'NONE', #12611, 1.500000000000003997 ) ;
#6232=EDGE_CURVE ( 'NONE', #6390, #9536, #11520, .T. ) ;
#6234=CYLINDRICAL_SURFACE ( 'NONE', #5356, 1.499999999999997780 ) ;
#6251=CARTESIAN_POINT ( 'NONE',  ( 8.883544964651964193, 0.000000000000000000, -12.08646469655236544 ) ) ;
#6254=CARTESIAN_POINT ( 'NONE',  ( -12.08646469655240097, 3.000000000000000000, -8.883544964651921561 ) ) ;
#6260=ORIENTED_EDGE ( 'NONE', *, *, #2980, .F. ) ;
#6262=ADVANCED_FACE ( 'NONE', ( #4796 ), #13197, .T. ) ;
#6263=VERTEX_POINT ( 'NONE', #3895 ) ;
#6269=CARTESIAN_POINT ( 'NONE',  ( -9.375397774054503586, 0.000000000000000000, -11.70905276178452503 ) ) ;
#6278=B_SPLINE_CURVE_WITH_KNOTS ( 'NONE', 3,
 ( #4162, #1972, #9589, #13475 ),
 .UNSPECIFIED., .F., .F.,
 ( 4, 4 ),
 ( 0.5454515525569062495, 0.5748696296145745510 ),
 .UNSPECIFIED. ) ;
#6281=B_SPLINE_CURVE_WITH_KNOTS ( 'NONE', 2,
 ( #11104, #8807, #13104 ),
 .UNSPECIFIED., .F., .F.,
 ( 3, 3 ),
 ( 0.000000000000000000, 0.02941149433826504428 ),
 .UNSPECIFIED. ) ;
#6282=CARTESIAN_POINT ( 'NONE',  ( -8.795158114916672432, 3.000000000000000000, -9.573149624528774382 ) ) ;
#6284=FACE_OUTER_BOUND ( 'NONE', #12168, .T. ) ;
#6285=CARTESIAN_POINT ( 'NONE',  ( -11.63517940784383775, 0.000000000000000000, -7.494008246337203083 ) ) ;
#6294=ORIENTED_EDGE ( 'NONE', *, *, #8096, .F. ) ;
#6296=ORIENTED_EDGE ( 'NONE', *, *, #857, .F. ) ;
#6298=CARTESIAN_POINT ( 'NONE',  ( 6.017756925049591921, 3.000000000000000000, -11.52330688609011844 ) ) ;
#6310=B_SPLINE_SURFACE_WITH_KNOTS ( 'NONE', 3, 1, ( 
 ( #6335, #6269 ),
 ( #1039, #12618 ),
 ( #4971, #13445 ),
 ( #3926, #12496 ) ),
 .UNSPECIFIED., .F., .F., .F.,
 ( 4, 4 ),
 ( 2, 2 ),
 ( 0.000000000000000000, 0.5855695330273008592 ),
 ( 0.000000000000000000, 1.000000000000000000 ),
 .UNSPECIFIED. ) ;
#6315=CARTESIAN_POINT ( 'NONE',  ( 7.494008246337245716, 3.000000000000000000, -11.63517940784380578 ) ) ;
#6317=DIRECTION ( 'NONE',  ( -0.000000000000000000, -1.000000000000000000, -0.000000000000000000 ) ) ;
#6323=ORIENTED_EDGE ( 'NONE', *, *, #13471, .T. ) ;
#6333=CARTESIAN_POINT ( 'NONE',  ( 30.73000000000000043, 3.000000000000000000, -3.999999999999999112 ) ) ;
#6335=CARTESIAN_POINT ( 'NONE',  ( -9.375397774054503586, 3.000000000000000000, -11.70905276178452503 ) ) ;
#6337=ADVANCED_FACE ( 'NONE', ( #5337 ), #4166, .T. ) ;
#6339=CARTESIAN_POINT ( 'NONE',  ( 1.958311002203130480, 0.000000000000000000, -14.87484884897977366 ) ) ;
#6340=VERTEX_POINT ( 'NONE', #1140 ) ;
#6342=ORIENTED_EDGE ( 'NONE', *, *, #5506, .T. ) ;
#6345=CARTESIAN_POINT ( 'NONE',  ( -4.821006024661084410, 0.000000000000000000, -13.61374091949017640 ) ) ;
#6350=CARTESIAN_POINT ( 'NONE',  ( 5.452638258930520010, 3.000000000000000000, -13.97385902380752754 ) ) ;
#6353=EDGE_CURVE ( 'NONE', #8307, #3554, #4298, .T. ) ;
#6359=ORIENTED_EDGE ( 'NONE', *, *, #7784, .F. ) ;
#6368=CARTESIAN_POINT ( 'NONE',  ( -11.52330688609014686, 3.000000000000000000, -6.017756925049552841 ) ) ;
#6371=ORIENTED_EDGE ( 'NONE', *, *, #6763, .T. ) ;
#6376=CIRCLE ( 'NONE', #13430, 1.000000000000001776 ) ;
#6390=VERTEX_POINT ( 'NONE', #2043 ) ;
#6402=FACE_OUTER_BOUND ( 'NONE', #786, .T. ) ;
#6405=VERTEX_POINT ( 'NONE', #5268 ) ;
#6407=EDGE_LOOP ( 'NONE', ( #9414, #2628 ) ) ;
#6414=DIRECTION ( 'NONE',  ( 0.000000000000000000, 0.000000000000000000, 1.000000000000000000 ) ) ;
#6428=B_SPLINE_SURFACE_WITH_KNOTS ( 'NONE', 3, 1, ( 
 ( #9656, #3514 ),
 ( #232, #8609 ),
 ( #12836, #5588 ),
 ( #10826, #2220 ) ),
 .UNSPECIFIED., .F., .F., .F.,
 ( 4, 4 ),
 ( 2, 2 ),
 ( 0.000000000000000000, 0.5855695330273008592 ),
 ( 0.000000000000000000, 1.000000000000000000 ),
 .UNSPECIFIED. ) ;
#6430=VERTEX_POINT ( 'NONE', #5672 ) ;
#6453=CIRCLE ( 'NONE', #516, 1.499999999999997780 ) ;
#6456=CARTESIAN_POINT ( 'NONE',  ( 10.97318381393774089, 3.000000000000000000, -6.970598036433387712 ) ) ;
#6457=CARTESIAN_POINT ( 'NONE',  ( -4.227250083625790467, 0.000000000000000000, -13.17831234185026013 ) ) ;
#6473=CARTESIAN_POINT ( 'NONE',  ( 4.821006024660968947, 0.000000000000000000, -13.61374091949021015 ) ) ;
#6475=CARTESIAN_POINT ( 'NONE',  ( -2.264806262022998062, 3.000000000000000000, -14.82803603298499340 ) ) ;
#6477=CARTESIAN_POINT ( 'NONE',  ( -13.97385902380755240, 0.000000000000000000, -5.452638258930474713 ) ) ;
#6481=VERTEX_POINT ( 'NONE', #9737 ) ;
#6483=CIRCLE ( 'NONE', #772, 12.99999999999977973 ) ;
#6489=DIRECTION ( 'NONE',  ( -0.000000000000000000, -1.000000000000000000, -0.000000000000000000 ) ) ;
#6491=CARTESIAN_POINT ( 'NONE',  ( -8.883544964652065445, 0.000000000000000000, -12.08646469655229438 ) ) ;
#6499=CARTESIAN_POINT ( 'NONE',  ( 3.893011711613070691, 3.000000000000000000, -12.40340517008307231 ) ) ;
#6506=ADVANCED_FACE ( 'NONE', ( #11677 ), #11419, .F. ) ;
#6507=CARTESIAN_POINT ( 'NONE',  ( 12.57851281883977457, 3.000000000000000000, 3.283445639306028063 ) ) ;
#6510=CARTESIAN_POINT ( 'NONE',  ( -1.958311002203252160, 3.000000000000000000, -14.87484884897975768 ) ) ;
#6515=ORIENTED_EDGE ( 'NONE', *, *, #13551, .T. ) ;
#6523=CARTESIAN_POINT ( 'NONE',  ( -4.821006024661084410, 0.000000000000000000, -13.61374091949017640 ) ) ;
#6527=CARTESIAN_POINT ( 'NONE',  ( 6.025412986832064277, 0.000000000000000000, -13.73660796332615597 ) ) ;
#6528=EDGE_CURVE ( 'NONE', #4567, #12679, #10847, .T. ) ;
#6533=ORIENTED_EDGE ( 'NONE', *, *, #888, .T. ) ;
#6539=( NAMED_UNIT ( * ) PLANE_ANGLE_UNIT ( ) SI_UNIT ( $, .RADIAN. ) );
#6543=FACE_OUTER_BOUND ( 'NONE', #622, .T. ) ;
#6545=CARTESIAN_POINT ( 'NONE',  ( 10.97318381393774089, 0.000000000000000000, -6.970598036433387712 ) ) ;
#6557=CARTESIAN_POINT ( 'NONE',  ( 0.000000000000000000, 0.000000000000000000, 0.000000000000000000 ) ) ;
#6574=CARTESIAN_POINT ( 'NONE',  ( 2.830255545554135832, 3.000000000000000000, -12.68816982652952596 ) ) ;
#6580=CARTESIAN_POINT ( 'NONE',  ( -12.40347894490204794, 3.000000000000000000, 3.892776652129663173 ) ) ;
#6604=EDGE_CURVE ( 'NONE', #11919, #1456, #13337, .T. ) ;
#6606=CARTESIAN_POINT ( 'NONE',  ( 8.883544964651964193, 0.000000000000000000, -12.08646469655236544 ) ) ;
#6615=LINE ( 'NONE', #13095, #942 ) ;
#6625=FACE_OUTER_BOUND ( 'NONE', #6127, .T. ) ;
#6632=ORIENTED_EDGE ( 'NONE', *, *, #10323, .F. ) ;
#6652=CARTESIAN_POINT ( 'NONE',  ( -6.017756925049793537, 3.000000000000000000, -11.52330688609026232 ) ) ;
#6653=AXIS2_PLACEMENT_3D ( 'NONE', #5109, #7315, #10418 ) ;
#6666=EDGE_LOOP ( 'NONE', ( #4852, #430 ) ) ;
#6682=CARTESIAN_POINT ( 'NONE',  ( -12.40340517008309185, 0.000000000000000000, -3.893011711613028947 ) ) ;
#6696=LINE ( 'NONE', #8685, #10217 ) ;
#6700=CARTESIAN_POINT ( 'NONE',  ( 6.970598036433451661, 0.000000000000000000, -10.97318381393796294 ) ) ;
#6705=VERTEX_POINT ( 'NONE', #4215 ) ;
#6712=DIRECTION ( 'NONE',  ( -0.000000000000000000, -1.000000000000000000, -0.000000000000000000 ) ) ;
#6720=CARTESIAN_POINT ( 'NONE',  ( -14.82803603298498629, 0.000000000000000000, 2.264806262023049577 ) ) ;
#6730=VERTEX_POINT ( 'NONE', #13537 ) ;
#6740=ADVANCED_FACE ( 'NONE', ( #999 ), #13466, .F. ) ;
#6743=CARTESIAN_POINT ( 'NONE',  ( 6.017756925049591921, 3.000000000000000000, -11.52330688609011844 ) ) ;
#6744=ORIENTED_EDGE ( 'NONE', *, *, #2114, .F. ) ;
#6746=CARTESIAN_POINT ( 'NONE',  ( -2.264806262022998062, 0.000000000000000000, -14.82803603298499340 ) ) ;
#6750=CARTESIAN_POINT ( 'NONE',  ( -14.82803603298498629, 3.000000000000000000, 2.264806262023049577 ) ) ;
#6752=ORIENTED_EDGE ( 'NONE', *, *, #2483, .F. ) ;
#6754=CARTESIAN_POINT ( 'NONE',  ( 0.000000000000000000, 0.000000000000000000, 0.000000000000000000 ) ) ;
#6757=CARTESIAN_POINT ( 'NONE',  ( 9.375397774054407662, 0.000000000000000000, -11.70905276178460497 ) ) ;
#6763=EDGE_CURVE ( 'NONE', #3554, #12628, #8286, .T. ) ;
#6766=B_SPLINE_CURVE_WITH_KNOTS ( 'NONE', 2,
 ( #7260, #8411, #5049 ),
 .UNSPECIFIED., .F., .F.,
 ( 3, 3 ),
 ( 0.000000000000000000, 1.000000000000000000 ),
 .UNSPECIFIED. ) ;
#6769=CARTESIAN_POINT ( 'NONE',  ( -1.650143266773857142, 3.000000000000000000, -14.90895795148409952 ) ) ;
#6772=ADVANCED_FACE ( 'NONE', ( #10231 ), #4745, .F. ) ;
#6795=ORIENTED_EDGE ( 'NONE', *, *, #1359, .F. ) ;
#6828=VERTEX_POINT ( 'NONE', #3388 ) ;
#6831=B_SPLINE_SURFACE_WITH_KNOTS ( 'NONE', 2, 1, ( 
 ( #207, #2398 ),
 ( #8928, #11281 ),
 ( #5692, #9966 ) ),
 .UNSPECIFIED., .F., .F., .F.,
 ( 3, 3 ),
 ( 2, 2 ),
 ( 0.000000000000000000, 1.000000000000000000 ),
 ( 0.000000000000000000, 1.000000000000000000 ),
 .UNSPECIFIED. ) ;
#6839=CARTESIAN_POINT ( 'NONE',  ( -6.970598036433426792, 3.000000000000000000, -10.97318381393771780 ) ) ;
#6861=DIRECTION ( 'NONE',  ( 0.000000000000000000, 1.000000000000000000, 0.000000000000000000 ) ) ;
#6867=VERTEX_POINT ( 'NONE', #1322 ) ;
#6871=CIRCLE ( 'NONE', #4885, 1.500000000000000666 ) ;
#6879=CARTESIAN_POINT ( 'NONE',  ( 30.66173999750687784, 3.000000000000000000, 0.01003121477750366919 ) ) ;
#6880=ORIENTED_EDGE ( 'NONE', *, *, #9876, .F. ) ;
#6890=CARTESIAN_POINT ( 'NONE',  ( -13.03533457366735426, 3.000000000000000000, -6.217402469309218027 ) ) ;
#6896=CARTESIAN_POINT ( 'NONE',  ( -3.188443695493920593, 0.000000000000000000, -12.60833606734848189 ) ) ;
#6900=ORIENTED_EDGE ( 'NONE', *, *, #2101, .F. ) ;
#6934=EDGE_CURVE ( 'NONE', #10001, #9552, #1195, .T. ) ;
#6944=ORIENTED_EDGE ( 'NONE', *, *, #9677, .F. ) ;
#6949=( GEOMETRIC_REPRESENTATION_CONTEXT ( 3 ) GLOBAL_UNCERTAINTY_ASSIGNED_CONTEXT ( ( #8737 ) ) GLOBAL_UNIT_ASSIGNED_CONTEXT ( ( #9898, #8662, #2401 ) ) REPRESENTATION_CONTEXT ( 'NONE', 'WORKASPACE' ) );
#6961=ORIENTED_EDGE ( 'NONE', *, *, #9677, .T. ) ;
#6965=EDGE_LOOP ( 'NONE', ( #4, #5037, #12699, #5630 ) ) ;
#6967=ORIENTED_EDGE ( 'NONE', *, *, #12254, .T. ) ;
#6976=CARTESIAN_POINT ( 'NONE',  ( -6.025412986832177076, 0.000000000000000000, -13.73660796332610268 ) ) ;
#6978=B_SPLINE_CURVE_WITH_KNOTS ( 'NONE', 3,
 ( #8195, #2827, #5999, #12429 ),
 .UNSPECIFIED., .F., .F.,
 ( 4, 4 ),
 ( 0.4545418633443863987, 0.4839599404020549223 ),
 .UNSPECIFIED. ) ;
#6981=ORIENTED_EDGE ( 'NONE', *, *, #12742, .T. ) ;
#6984=CARTESIAN_POINT ( 'NONE',  ( 9.573149624528804580, 3.000000000000000000, -8.795158114916638681 ) ) ;
#6987=DIRECTION ( 'NONE',  ( -0.9893737785712105604, -0.000000000000000000, 0.1453943818575021141 ) ) ;
#6996=ORIENTED_EDGE ( 'NONE', *, *, #2101, .T. ) ;
#6997=ORIENTED_EDGE ( 'NONE', *, *, #4725, .T. ) ;
#7003=CARTESIAN_POINT ( 'NONE',  ( -14.82803603298498629, 0.000000000000000000, 2.264806262023049577 ) ) ;
#7013=CARTESIAN_POINT ( 'NONE',  ( 1.958311002203130480, 0.000000000000000000, -14.87484884897977366 ) ) ;
#7016=CARTESIAN_POINT ( 'NONE',  ( -10.98198414889942676, 0.000000000000000000, -9.379342464487661957 ) ) ;
#7018=EDGE_CURVE ( 'NONE', #8307, #4532, #13238, .T. ) ;
#7028=CARTESIAN_POINT ( 'NONE',  ( 11.59535436762926430, 0.000000000000000000, -5.877734009726468756 ) ) ;
#7032=CARTESIAN_POINT ( 'NONE',  ( -6.025412986832177076, 0.000000000000000000, -13.73660796332610268 ) ) ;
#7038=FACE_OUTER_BOUND ( 'NONE', #5594, .T. ) ;
#7042=CARTESIAN_POINT ( 'NONE',  ( -6.329356821613726147, 0.000000000000000000, -12.30759122142001338 ) ) ;
#7056=CARTESIAN_POINT ( 'NONE',  ( 9.133371500908369356, 3.000000000000000000, -11.90284147956862171 ) ) ;
#7067=ORIENTED_EDGE ( 'NONE', *, *, #3782, .T. ) ;
#7076=ADVANCED_FACE ( 'NONE', ( #4828 ), #10833, .F. ) ;
#7091=ADVANCED_FACE ( 'NONE', ( #7038 ), #9499, .F. ) ;
#7093=CARTESIAN_POINT ( 'NONE',  ( -11.35348746973813761, 3.000000000000000000, -6.343077501554963860 ) ) ;
#7110=DIRECTION ( 'NONE',  ( 0.000000000000000000, 1.000000000000000000, 0.000000000000000000 ) ) ;
#7116=CARTESIAN_POINT ( 'NONE',  ( 8.795158114916441505, 3.000000000000000000, -9.573149624528689117 ) ) ;
#7130=LINE ( 'NONE', #6219, #8353 ) ;
#7133=EDGE_CURVE ( 'NONE', #12719, #3825, #5552, .T. ) ;
#7137=CIRCLE ( 'NONE', #1188, 1.500000000000003997 ) ;
#7144=VERTEX_POINT ( 'NONE', #12498 ) ;
#7164=CARTESIAN_POINT ( 'NONE',  ( -9.375397774054503586, 3.000000000000000000, -11.70905276178452503 ) ) ;
#7172=STYLED_ITEM ( 'NONE', ( #8727 ), #2434 ) ;
#7185=CARTESIAN_POINT ( 'NONE',  ( 9.375397774054407662, 0.000000000000000000, -11.70905276178460497 ) ) ;
#7205=CARTESIAN_POINT ( 'NONE',  ( -11.35348746973813761, 3.000000000000000000, -6.343077501554963860 ) ) ;
#7207=VERTEX_POINT ( 'NONE', #11710 ) ;
#7209=EDGE_CURVE ( 'NONE', #13403, #2130, #12692, .T. ) ;
#7211=ORIENTED_EDGE ( 'NONE', *, *, #2114, .T. ) ;
#7214=PLANE ( 'NONE',  #254 ) ;
#7234=EDGE_CURVE ( 'NONE', #11204, #2891, #1286, .T. ) ;
#7237=B_SPLINE_CURVE_WITH_KNOTS ( 'NONE', 2,
 ( #5044, #10496, #11527 ),
 .UNSPECIFIED., .F., .F.,
 ( 3, 3 ),
 ( 0.000000000000000000, 1.000000000000000000 ),
 .UNSPECIFIED. ) ;
#7242=CARTESIAN_POINT ( 'NONE',  ( 1.650143266773734796, 3.000000000000000000, -14.90895795148410841 ) ) ;
#7260=CARTESIAN_POINT ( 'NONE',  ( -14.82803603298502360, 0.000000000000000000, -2.264806262022826644 ) ) ;
#7276=DIRECTION ( 'NONE',  ( -0.000000000000000000, -1.000000000000000000, 0.000000000000000000 ) ) ;
#7279=CARTESIAN_POINT ( 'NONE',  ( -13.03533457366735426, 3.000000000000000000, -6.217402469309218027 ) ) ;
#7282=B_SPLINE_SURFACE_WITH_KNOTS ( 'NONE', 3, 1, ( 
 ( #2591, #9200 ),
 ( #3832, #13409 ),
 ( #9136, #8033 ),
 ( #1640, #3962 ) ),
 .UNSPECIFIED., .F., .F., .F.,
 ( 4, 4 ),
 ( 2, 2 ),
 ( 0.000000000000000000, 0.5855695330273008592 ),
 ( 0.000000000000000000, 1.000000000000000000 ),
 .UNSPECIFIED. ) ;
#7286=VECTOR ( 'NONE', #551, 1000.000000000000000 ) ;
#7296=DIRECTION ( 'NONE',  ( -0.000000000000000000, -1.000000000000000000, -0.000000000000000000 ) ) ;
#7300=CARTESIAN_POINT ( 'NONE',  ( 0.5501230721522984979, 0.000000000000000000, -12.98835496148321766 ) ) ;
#7305=CARTESIAN_POINT ( 'NONE',  ( -13.73660796332618261, 0.000000000000000000, -6.025412986832017204 ) ) ;
#7308=B_SPLINE_CURVE_WITH_KNOTS ( 'NONE', 3,
 ( #5540, #2444, #4443, #3410 ),
 .UNSPECIFIED., .F., .F.,
 ( 4, 4 ),
 ( 0.000000000000000000, 0.5855695330273008592 ),
 .UNSPECIFIED. ) ;
#7315=DIRECTION ( 'NONE',  ( 0.000000000000000000, 1.000000000000000000, 0.000000000000000000 ) ) ;
#7316=ORIENTED_EDGE ( 'NONE', *, *, #1288, .T. ) ;
#7320=VECTOR ( 'NONE', #4285, 1000.000000000000000 ) ;
#7322=CARTESIAN_POINT ( 'NONE',  ( 12.08646469655232636, 0.000000000000000000, -8.883544964652022813 ) ) ;
#7329=ORIENTED_EDGE ( 'NONE', *, *, #7018, .F. ) ;
#7337=ORIENTED_EDGE ( 'NONE', *, *, #13267, .T. ) ;
#7359=CARTESIAN_POINT ( 'NONE',  ( 11.70905276178455878, 0.000000000000000000, -9.375397774054460953 ) ) ;
#7363=EDGE_CURVE ( 'NONE', #5524, #4532, #4583, .T. ) ;
#7364=LINE ( 'NONE', #1992, #1886 ) ;
#7380=CARTESIAN_POINT ( 'NONE',  ( -2.264806262022998062, 3.000000000000000000, -14.82803603298499340 ) ) ;
#7382=LINE ( 'NONE', #8327, #12871 ) ;
#7391=CARTESIAN_POINT ( 'NONE',  ( 30.73000000000000043, 0.000000000000000000, -3.999999999999999112 ) ) ;
#7403=CARTESIAN_POINT ( 'NONE',  ( -11.52330688609014686, 3.000000000000000000, -6.017756925049552841 ) ) ;
#7416=EDGE_CURVE ( 'NONE', #5310, #3210, #274, .T. ) ;
#7420=EDGE_LOOP ( 'NONE', ( #3436, #10638, #1031, #4029 ) ) ;
#7422=EDGE_CURVE ( 'NONE', #8734, #12207, #3639, .T. ) ;
#7432=ORIENTED_EDGE ( 'NONE', *, *, #11466, .F. ) ;
#7438=B_SPLINE_SURFACE_WITH_KNOTS ( 'NONE', 3, 1, ( 
 ( #10524, #6251 ),
 ( #1083, #3146 ),
 ( #6315, #2181 ),
 ( #10464, #4324 ) ),
 .UNSPECIFIED., .F., .F., .F.,
 ( 4, 4 ),
 ( 2, 2 ),
 ( 0.000000000000000000, 0.5855695330273008592 ),
 ( 0.000000000000000000, 1.000000000000000000 ),
 .UNSPECIFIED. ) ;
#7442=CARTESIAN_POINT ( 'NONE',  ( -8.883544964652065445, 0.000000000000000000, -12.08646469655229438 ) ) ;
#7443=CARTESIAN_POINT ( 'NONE',  ( 9.375397774054407662, 0.000000000000000000, -11.70905276178460497 ) ) ;
#7444=CARTESIAN_POINT ( 'NONE',  ( -10.98198414889942676, 0.000000000000000000, -9.379342464487661957 ) ) ;
#7450=EDGE_CURVE ( 'NONE', #12351, #9536, #4812, .T. ) ;
#7457=CARTESIAN_POINT ( 'NONE',  ( -12.60833596047604210, 3.000000000000000000, -3.188441730140805674 ) ) ;
#7460=DIRECTION ( 'NONE',  ( 0.000000000000000000, -1.000000000000000000, 0.000000000000000000 ) ) ;
#7462=CARTESIAN_POINT ( 'NONE',  ( -9.324917476840782982, 3.000000000000000000, -9.065441278446241924 ) ) ;
#7466=ORIENTED_EDGE ( 'NONE', *, *, #12219, .F. ) ;
#7467=EDGE_CURVE ( 'NONE', #3538, #9896, #11488, .T. ) ;
#7470=AXIS2_PLACEMENT_3D ( 'NONE', #4806, #1718, #137 ) ;
#7477=ORIENTED_EDGE ( 'NONE', *, *, #12349, .T. ) ;
#7480=ORIENTED_EDGE ( 'NONE', *, *, #49, .F. ) ;
#7489=CARTESIAN_POINT ( 'NONE',  ( -13.86115248177182835, 3.000000000000000000, -5.741477348071267528 ) ) ;
#7490=CARTESIAN_POINT ( 'NONE',  ( 0.000000000000000000, 3.000000000000000000, -1.500000000000000222 ) ) ;
#7492=ORIENTED_EDGE ( 'NONE', *, *, #13582, .F. ) ;
#7514=EDGE_LOOP ( 'NONE', ( #5275, #2559, #5986, #12081 ) ) ;
#7515=VERTEX_POINT ( 'NONE', #11679 ) ;
#7529=ORIENTED_EDGE ( 'NONE', *, *, #8008, .F. ) ;
#7531=PRODUCT ( 'gear-link-2', 'gear-link-2', '', ( #10770 ) ) ;
#7553=CARTESIAN_POINT ( 'NONE',  ( -14.90895795148411374, 3.000000000000000000, -1.650143266773683726 ) ) ;
#7558=DIRECTION ( 'NONE',  ( -0.000000000000000000, -1.000000000000000000, -0.000000000000000000 ) ) ;
#7560=LINE ( 'NONE', #2124, #12650 ) ;
#7569=ADVANCED_FACE ( 'NONE', ( #5984 ), #2471, .F. ) ;
#7573=SURFACE_STYLE_USAGE ( .BOTH. , #1239 ) ;
#7587=DIRECTION ( 'NONE',  ( -0.000000000000000000, -1.000000000000000000, -0.000000000000000000 ) ) ;
#7591=CARTESIAN_POINT ( 'NONE',  ( 8.795158114916441505, 3.000000000000000000, -9.573149624528689117 ) ) ;
#7592=EDGE_CURVE ( 'NONE', #11130, #7605, #13023, .T. ) ;
#7594=B_SPLINE_CURVE_WITH_KNOTS ( 'NONE', 3,
 ( #9529, #4294, #7462, #2222 ),
 .UNSPECIFIED., .F., .F.,
 ( 4, 4 ),
 ( 0.3636321741318673806, 0.3930502511895355711 ),
 .UNSPECIFIED. ) ;
#7600=VECTOR ( 'NONE', #4477, 1000.000000000000000 ) ;
#7605=VERTEX_POINT ( 'NONE', #4577 ) ;
#7613=CARTESIAN_POINT ( 'NONE',  ( 0.6724118135762067183, 0.000000000000000000, -13.82336506795094344 ) ) ;
#7614=DIRECTION ( 'NONE',  ( 0.000000000000000000, 0.000000000000000000, -1.000000000000000000 ) ) ;
#7631=CARTESIAN_POINT ( 'NONE',  ( 3.893011711613070691, 0.000000000000000000, -12.40340517008307231 ) ) ;
#7636=ORIENTED_EDGE ( 'NONE', *, *, #10798, .T. ) ;
#7639=CARTESIAN_POINT ( 'NONE',  ( -5.741477348071430065, 0.000000000000000000, -13.86115248177175374 ) ) ;
#7644=CARTESIAN_POINT ( 'NONE',  ( 12.08646469655232636, 0.000000000000000000, -8.883544964652022813 ) ) ;
#7647=ORIENTED_EDGE ( 'NONE', *, *, #4100, .F. ) ;
#7652=ORIENTED_EDGE ( 'NONE', *, *, #842, .F. ) ;
#7654=CARTESIAN_POINT ( 'NONE',  ( -13.03533457366735426, 0.000000000000000000, -6.217402469309218027 ) ) ;
#7659=CARTESIAN_POINT ( 'NONE',  ( -13.82336506795071607, 0.000000000000000000, 0.6724118135763649251 ) ) ;
#7661=ORIENTED_EDGE ( 'NONE', *, *, #10798, .F. ) ;
#7675=EDGE_CURVE ( 'NONE', #2426, #3437, #4559, .T. ) ;
#7682=CARTESIAN_POINT ( 'NONE',  ( 8.180229652970799847, 3.000000000000000000, -11.90209577080762848 ) ) ;
#7686=DIRECTION ( 'NONE',  ( 0.000000000000000000, 0.000000000000000000, -1.000000000000000000 ) ) ;
#7692=ORIENTED_EDGE ( 'NONE', *, *, #8008, .T. ) ;
#7718=CARTESIAN_POINT ( 'NONE',  ( -13.82336506795094522, 3.000000000000000000, -0.6724118135761603110 ) ) ;
#7720=CARTESIAN_POINT ( 'NONE',  ( -14.82803603298502360, 3.000000000000000000, -2.264806262022826644 ) ) ;
#7729=ORIENTED_EDGE ( 'NONE', *, *, #11579, .F. ) ;
#7734=CARTESIAN_POINT ( 'NONE',  ( 11.70905276178455878, 0.000000000000000000, -9.375397774054460953 ) ) ;
#7740=VECTOR ( 'NONE', #11791, 1000.000000000000000 ) ;
#7741=ORIENTED_EDGE ( 'NONE', *, *, #6528, .F. ) ;
#7744=CARTESIAN_POINT ( 'NONE',  ( -5.452638258930639914, 0.000000000000000000, -13.97385902380748313 ) ) ;
#7760=CARTESIAN_POINT ( 'NONE',  ( -7.500000000000000000, 3.000000000000000000, 0.000000000000000000 ) ) ;
#7763=ORIENTED_EDGE ( 'NONE', *, *, #1854, .F. ) ;
#7766=B_SPLINE_CURVE_WITH_KNOTS ( 'NONE', 3,
 ( #4588, #1099, #5296, #4268 ),
 .UNSPECIFIED., .F., .F.,
 ( 4, 4 ),
 ( 0.000000000000000000, 0.5855695330273008592 ),
 .UNSPECIFIED. ) ;
#7778=DIRECTION ( 'NONE',  ( -0.9893737785712105604, 0.000000000000000000, 0.1453943818575020863 ) ) ;
#7784=EDGE_CURVE ( 'NONE', #9896, #8568, #12395, .T. ) ;
#7785=EDGE_CURVE ( 'NONE', #3437, #11402, #10084, .T. ) ;
#7789=CARTESIAN_POINT ( 'NONE',  ( 2.830255545554135832, 0.000000000000000000, -12.68816982652952596 ) ) ;
#7790=CARTESIAN_POINT ( 'NONE',  ( -13.82336506795094522, 0.000000000000000000, -0.6724118135761603110 ) ) ;
#7793=CARTESIAN_POINT ( 'NONE',  ( -14.82803603298502360, 3.000000000000000000, -2.264806262022826644 ) ) ;
#7797=CARTESIAN_POINT ( 'NONE',  ( -13.97385902380755240, 3.000000000000000000, -5.452638258930474713 ) ) ;
#7801=ORIENTED_EDGE ( 'NONE', *, *, #12254, .F. ) ;
#7806=CARTESIAN_POINT ( 'NONE',  ( -12.51336114795298471, 0.000000000000000000, -3.542894103880322998 ) ) ;
#7813=AXIS2_PLACEMENT_3D ( 'NONE', #2674, #763, #11013 ) ;
#7819=DIRECTION ( 'NONE',  ( -0.000000000000000000, -1.000000000000000000, -0.000000000000000000 ) ) ;
#7828=ORIENTED_EDGE ( 'NONE', *, *, #7133, .F. ) ;
#7836=CARTESIAN_POINT ( 'NONE',  ( 6.970598036433451661, 3.000000000000000000, -10.97318381393796294 ) ) ;
#7838=CARTESIAN_POINT ( 'NONE',  ( -13.97385902380755240, 3.000000000000000000, -5.452638258930474713 ) ) ;
#7839=CARTESIAN_POINT ( 'NONE',  ( -5.741477348071430065, 3.000000000000000000, -13.86115248177175374 ) ) ;
#7857=CARTESIAN_POINT ( 'NONE',  ( -6.217402469309367241, 0.000000000000000000, -13.03533457366727610 ) ) ;
#7860=VERTEX_POINT ( 'NONE', #4155 ) ;
#7866=FACE_OUTER_BOUND ( 'NONE', #13018, .T. ) ;
#7882=CARTESIAN_POINT ( 'NONE',  ( -0.5501230721523990841, 3.000000000000000000, -12.98835496148299384 ) ) ;
#7888=ORIENTED_EDGE ( 'NONE', *, *, #13323, .F. ) ;
#7889=ORIENTED_EDGE ( 'NONE', *, *, #12332, .T. ) ;
#7893=EDGE_CURVE ( 'NONE', #3759, #8307, #10141, .T. ) ;
#7900=CARTESIAN_POINT ( 'NONE',  ( -10.97318381393799136, 0.000000000000000000, -6.970598036433411693 ) ) ;
#7904=CARTESIAN_POINT ( 'NONE',  ( -7.500000000000000000, 3.000000000000000000, 0.000000000000000000 ) ) ;
#7923=DIRECTION ( 'NONE',  ( -0.000000000000000000, -1.000000000000000000, -0.000000000000000000 ) ) ;
#7936=DIRECTION ( 'NONE',  ( -0.000000000000000000, -1.000000000000000000, -0.000000000000000000 ) ) ;
#7940=CARTESIAN_POINT ( 'NONE',  ( -8.795158114916672432, 0.000000000000000000, -9.573149624528774382 ) ) ;
#7945=VECTOR ( 'NONE', #5336, 1000.000000000000000 ) ;
#7949=VERTEX_POINT ( 'NONE', #9250 ) ;
#7957=CARTESIAN_POINT ( 'NONE',  ( 6.970598036433451661, 0.000000000000000000, -10.97318381393796294 ) ) ;
#7958=B_SPLINE_CURVE_WITH_KNOTS ( 'NONE', 2,
 ( #2890, #9084, #9220 ),
 .UNSPECIFIED., .F., .F.,
 ( 3, 3 ),
 ( 0.000000000000000000, 1.000000000000000000 ),
 .UNSPECIFIED. ) ;
#7966=ORIENTED_EDGE ( 'NONE', *, *, #9632, .T. ) ;
#7968=CARTESIAN_POINT ( 'NONE',  ( 30.79786191028635400, 0.000000000000000000, -6.999232361977355765 ) ) ;
#7975=DIRECTION ( 'NONE',  ( -0.000000000000000000, -1.000000000000000000, -0.000000000000000000 ) ) ;
#7978=DIRECTION ( 'NONE',  ( 0.000000000000000000, 0.000000000000000000, 1.000000000000000000 ) ) ;
#7986=ORIENTED_EDGE ( 'NONE', *, *, #11810, .F. ) ;
#7988=ORIENTED_EDGE ( 'NONE', *, *, #6604, .T. ) ;
#7995=FACE_OUTER_BOUND ( 'NONE', #5092, .T. ) ;
#7996=FACE_OUTER_BOUND ( 'NONE', #9814, .T. ) ;
#8003=VERTEX_POINT ( 'NONE', #10565 ) ;
#8004=AXIS2_PLACEMENT_3D ( 'NONE', #4401, #8591, #3363 ) ;
#8008=EDGE_CURVE ( 'NONE', #12983, #7207, #1002, .T. ) ;
#8012=CARTESIAN_POINT ( 'NONE',  ( -12.98835496148299207, 0.000000000000000000, 0.5501230721524459355 ) ) ;
#8017=CARTESIAN_POINT ( 'NONE',  ( -9.573149624528719315, 3.000000000000000000, -8.795158114916407754 ) ) ;
#8033=CARTESIAN_POINT ( 'NONE',  ( -2.928250210355484828, 0.000000000000000000, -13.52637830886140335 ) ) ;
#8035=AXIS2_PLACEMENT_3D ( 'NONE', #4198, #12815, #2202 ) ;
#8056=EDGE_LOOP ( 'NONE', ( #7067, #13287, #305, #819 ) ) ;
#8059=UNCERTAINTY_MEASURE_WITH_UNIT (LENGTH_MEASURE( 1.000000000000000082E-05 ), #9635, 'distance_accuracy_value', 'NONE');
#8063=ORIENTED_EDGE ( 'NONE', *, *, #9275, .T. ) ;
#8068=CARTESIAN_POINT ( 'NONE',  ( 6.017756925049591921, 0.000000000000000000, -11.52330688609011844 ) ) ;
#8076=ORIENTED_EDGE ( 'NONE', *, *, #8995, .F. ) ;
#8083=ADVANCED_FACE ( 'NONE', ( #426 ), #2585, .F. ) ;
#8086=CARTESIAN_POINT ( 'NONE',  ( -6.017756925049793537, 3.000000000000000000, -11.52330688609026232 ) ) ;
#8091=ORIENTED_EDGE ( 'NONE', *, *, #7363, .T. ) ;
#8094=CARTESIAN_POINT ( 'NONE',  ( 7.499999999999999112, 3.000000000000000000, 0.000000000000000000 ) ) ;
#8096=EDGE_CURVE ( 'NONE', #5500, #12749, #11666, .T. ) ;
#8110=B_SPLINE_CURVE_WITH_KNOTS ( 'NONE', 2,
 ( #10091, #2935, #11199 ),
 .UNSPECIFIED., .F., .F.,
 ( 3, 3 ),
 ( 0.000000000000000000, 1.000000000000000000 ),
 .UNSPECIFIED. ) ;
#8116=CARTESIAN_POINT ( 'NONE',  ( 3.188443874008702661, 3.000000000000000000, -12.60833581801614578 ) ) ;
#8117=CARTESIAN_POINT ( 'NONE',  ( -11.17001009226120445, 0.000000000000000000, -6.660869730750943241 ) ) ;
#8119=CARTESIAN_POINT ( 'NONE',  ( -7.500000000000000000, 3.000000000000000000, -1.500000000000000666 ) ) ;
#8128=CARTESIAN_POINT ( 'NONE',  ( -0.6724118135763151871, 0.000000000000000000, -13.82336506795071784 ) ) ;
#8135=DIRECTION ( 'NONE',  ( -0.000000000000000000, -1.000000000000000000, 0.000000000000000000 ) ) ;
#8147=CARTESIAN_POINT ( 'NONE',  ( 11.90209577080759296, 3.000000000000000000, -8.180229652970856691 ) ) ;
#8151=VECTOR ( 'NONE', #7975, 1000.000000000000000 ) ;
#8157=EDGE_LOOP ( 'NONE', ( #5955, #12058, #8706, #9023 ) ) ;
#8163=FACE_OUTER_BOUND ( 'NONE', #1853, .T. ) ;
#8169=CARTESIAN_POINT ( 'NONE',  ( -4.227250083625790467, 3.000000000000000000, -13.17831234185026013 ) ) ;
#8174=AXIS2_PLACEMENT_3D ( 'NONE', #9553, #3265, #134 ) ;
#8179=CARTESIAN_POINT ( 'NONE',  ( -11.90284147956865723, 3.000000000000000000, -9.133371500908332052 ) ) ;
#8184=VERTEX_POINT ( 'NONE', #10213 ) ;
#8193=EDGE_CURVE ( 'NONE', #3554, #8734, #3716, .T. ) ;
#8195=CARTESIAN_POINT ( 'NONE',  ( -6.017756925049793537, 0.000000000000000000, -11.52330688609026232 ) ) ;
#8227=DIRECTION ( 'NONE',  ( 0.000000000000000000, 1.000000000000000000, 0.000000000000000000 ) ) ;
#8228=AXIS2_PLACEMENT_3D ( 'NONE', #10596, #1157, #5355 ) ;
#8231=B_SPLINE_CURVE_WITH_KNOTS ( 'NONE', 2,
 ( #10320, #8179, #6254 ),
 .UNSPECIFIED., .F., .F.,
 ( 3, 3 ),
 ( 0.000000000000000000, 1.000000000000000000 ),
 .UNSPECIFIED. ) ;
#8246=FACE_OUTER_BOUND ( 'NONE', #5024, .T. ) ;
#8249=EDGE_CURVE ( 'NONE', #1536, #7207, #11782, .T. ) ;
#8255=CYLINDRICAL_SURFACE ( 'NONE', #2541, 1.000000000000000888 ) ;
#8264=CARTESIAN_POINT ( 'NONE',  ( -14.82803603298498629, 3.000000000000000000, 2.264806262023049577 ) ) ;
#8268=FACE_OUTER_BOUND ( 'NONE', #11721, .T. ) ;
#8270=CARTESIAN_POINT ( 'NONE',  ( 1.958311002203130480, 3.000000000000000000, -14.87484884897977366 ) ) ;
#8273=DIRECTION ( 'NONE',  ( 0.000000000000000000, 0.000000000000000000, -1.000000000000000000 ) ) ;
#8276=ORIENTED_EDGE ( 'NONE', *, *, #10057, .T. ) ;
#8286=LINE ( 'NONE', #9183, #4649 ) ;
#8291=ORIENTED_EDGE ( 'NONE', *, *, #5806, .T. ) ;
#8294=ORIENTED_EDGE ( 'NONE', *, *, #3782, .F. ) ;
#8299=CARTESIAN_POINT ( 'NONE',  ( 30.66173999750687784, 0.000000000000000000, 0.01003121477750366919 ) ) ;
#8306=B_SPLINE_CURVE_WITH_KNOTS ( 'NONE', 3,
 ( #6746, #10949, #12606, #6190 ),
 .UNSPECIFIED., .F., .F.,
 ( 4, 4 ),
 ( 0.000000000000000000, 0.5855695330273008592 ),
 .UNSPECIFIED. ) ;
#8307=VERTEX_POINT ( 'NONE', #6206 ) ;
#8312=CARTESIAN_POINT ( 'NONE',  ( 10.25006213149504752, 3.000000000000000000, -9.299128225235653744 ) ) ;
#8315=FACE_OUTER_BOUND ( 'NONE', #11428, .T. ) ;
#8317=ORIENTED_EDGE ( 'NONE', *, *, #10459, .F. ) ;
#8319=EDGE_CURVE ( 'NONE', #8184, #1339, #8843, .T. ) ;
#8326=CARTESIAN_POINT ( 'NONE',  ( 8.795158114916441505, 0.000000000000000000, -9.573149624528689117 ) ) ;
#8327=CARTESIAN_POINT ( 'NONE',  ( 13.40069634612381044, 3.000000000000000000, 2.546644602219900300 ) ) ;
#8330=ORIENTED_EDGE ( 'NONE', *, *, #4202, .F. ) ;
#8344=DIRECTION ( 'NONE',  ( -0.000000000000000000, -1.000000000000000000, -0.000000000000000000 ) ) ;
#8345=CARTESIAN_POINT ( 'NONE',  ( 10.97318381393774089, 0.000000000000000000, -6.970598036433387712 ) ) ;
#8347=VERTEX_POINT ( 'NONE', #13520 ) ;
#8350=VERTEX_POINT ( 'NONE', #12362 ) ;
#8353=VECTOR ( 'NONE', #12567, 1000.000000000000000 ) ;
#8358=CARTESIAN_POINT ( 'NONE',  ( 12.48730470360076161, 0.000000000000000000, -6.329867395090054139 ) ) ;
#8363=VECTOR ( 'NONE', #5494, 1000.000000000000000 ) ;
#8379=FACE_OUTER_BOUND ( 'NONE', #1029, .T. ) ;
#8390=CARTESIAN_POINT ( 'NONE',  ( 4.227250083625740729, 0.000000000000000000, -13.17831234185050526 ) ) ;
#8391=CARTESIAN_POINT ( 'NONE',  ( 0.5501230721522984979, 0.000000000000000000, -12.98835496148321766 ) ) ;
#8407=VECTOR ( 'NONE', #13399, 1000.000000000000000 ) ;
#8411=CARTESIAN_POINT ( 'NONE',  ( -14.87484884897978077, 0.000000000000000000, -1.958311002203079187 ) ) ;
#8412=B_SPLINE_SURFACE_WITH_KNOTS ( 'NONE', 3, 1, ( 
 ( #4512, #3670 ),
 ( #5608, #8906 ),
 ( #12029, #1272 ),
 ( #4640, #4575 ) ),
 .UNSPECIFIED., .F., .F., .F.,
 ( 4, 4 ),
 ( 2, 2 ),
 ( 0.3636321741318673806, 0.3930502511895355711 ),
 ( 0.000000000000000000, 1.000000000000000000 ),
 .UNSPECIFIED. ) ;
#8432=DIRECTION ( 'NONE',  ( 0.000000000000000000, 0.000000000000000000, -1.000000000000000000 ) ) ;
#8433=CARTESIAN_POINT ( 'NONE',  ( 3.893011711613070691, 3.000000000000000000, -12.40340517008307231 ) ) ;
#8449=CARTESIAN_POINT ( 'NONE',  ( -13.97385902380755240, 0.000000000000000000, -5.452638258930474713 ) ) ;
#8474=ORIENTED_EDGE ( 'NONE', *, *, #11541, .F. ) ;
#8479=CARTESIAN_POINT ( 'NONE',  ( 9.573149624528804580, 3.000000000000000000, -8.795158114916638681 ) ) ;
#8481=CARTESIAN_POINT ( 'NONE',  ( -9.133371500908470608, 3.000000000000000000, -11.90284147956855065 ) ) ;
#8490=ORIENTED_EDGE ( 'NONE', *, *, #5171, .F. ) ;
#8492=CARTESIAN_POINT ( 'NONE',  ( -12.98835496148299207, 3.000000000000000000, 0.5501230721524459355 ) ) ;
#8495=DIRECTION ( 'NONE',  ( 0.000000000000000000, 0.000000000000000000, -1.000000000000000000 ) ) ;
#8498=CARTESIAN_POINT ( 'NONE',  ( 3.893011711613070691, 0.000000000000000000, -12.40340517008307231 ) ) ;
#8506=CARTESIAN_POINT ( 'NONE',  ( -12.56843238770841786, 3.000000000000000000, 3.367671042046304741 ) ) ;
#8510=CARTESIAN_POINT ( 'NONE',  ( -3.893011711613112880, 0.000000000000000000, -12.40340517008282717 ) ) ;
#8512=FACE_OUTER_BOUND ( 'NONE', #5151, .T. ) ;
#8514=CARTESIAN_POINT ( 'NONE',  ( 5.452638258930520010, 0.000000000000000000, -13.97385902380752754 ) ) ;
#8520=ORIENTED_EDGE ( 'NONE', *, *, #8193, .T. ) ;
#8525=CARTESIAN_POINT ( 'NONE',  ( -2.264806262022998062, 3.000000000000000000, -14.82803603298499340 ) ) ;
#8529=CARTESIAN_POINT ( 'NONE',  ( -8.883544964652065445, 3.000000000000000000, -12.08646469655229438 ) ) ;
#8540=CARTESIAN_POINT ( 'NONE',  ( -9.379342464487789854, 3.000000000000000000, -10.98198414889931307 ) ) ;
#8545=FACE_BOUND ( 'NONE', #10357, .T. ) ;
#8546=DIRECTION ( 'NONE',  ( -0.000000000000000000, -1.000000000000000000, -0.000000000000000000 ) ) ;
#8558=B_SPLINE_CURVE_WITH_KNOTS ( 'NONE', 3,
 ( #8510, #6457, #6523, #3218 ),
 .UNSPECIFIED., .F., .F.,
 ( 4, 4 ),
 ( 0.000000000000000000, 0.5855695330273008592 ),
 .UNSPECIFIED. ) ;
#8568=VERTEX_POINT ( 'NONE', #8872 ) ;
#8574=DIRECTION ( 'NONE',  ( 0.000000000000000000, 0.000000000000000000, 1.000000000000000000 ) ) ;
#8575=ADVANCED_FACE ( 'NONE', ( #5703 ), #5643, .F. ) ;
#8578=DIRECTION ( 'NONE',  ( 0.000000000000000000, 0.000000000000000000, 1.000000000000000000 ) ) ;
#8585=EDGE_CURVE ( 'NONE', #3916, #6405, #623, .T. ) ;
#8591=DIRECTION ( 'NONE',  ( 0.000000000000000000, 1.000000000000000000, 0.000000000000000000 ) ) ;
#8592=CARTESIAN_POINT ( 'NONE',  ( -1.958311002203252160, 0.000000000000000000, -14.87484884897975768 ) ) ;
#8595=CARTESIAN_POINT ( 'NONE',  ( 5.452638258930520010, 3.000000000000000000, -13.97385902380752754 ) ) ;
#8596=ORIENTED_EDGE ( 'NONE', *, *, #10020, .T. ) ;
#8598=ORIENTED_EDGE ( 'NONE', *, *, #3563, .T. ) ;
#8604=CARTESIAN_POINT ( 'NONE',  ( 9.065480927540312095, 3.000000000000000000, -9.324856600128422102 ) ) ;
#8608=VECTOR ( 'NONE', #3013, 1000.000000000000000 ) ;
#8609=CARTESIAN_POINT ( 'NONE',  ( 2.928250210355320959, 0.000000000000000000, -13.52637830886121506 ) ) ;
#8616=DIRECTION ( 'NONE',  ( -0.000000000000000000, -1.000000000000000000, -0.000000000000000000 ) ) ;
#8619=B_SPLINE_CURVE_WITH_KNOTS ( 'NONE', 3,
 ( #9851, #5714, #7790, #9991 ),
 .UNSPECIFIED., .F., .F.,
 ( 4, 4 ),
 ( 0.000000000000000000, 0.5855695330273008592 ),
 .UNSPECIFIED. ) ;
#8625=FACE_OUTER_BOUND ( 'NONE', #3570, .T. ) ;
#8627=FACE_OUTER_BOUND ( 'NONE', #6965, .T. ) ;
#8629=EDGE_CURVE ( 'NONE', #11917, #11340, #8306, .T. ) ;
#8638=FACE_OUTER_BOUND ( 'NONE', #2833, .T. ) ;
#8661=ADVANCED_FACE ( 'NONE', ( #8315 ), #4183, .F. ) ;
#8662=( NAMED_UNIT ( * ) PLANE_ANGLE_UNIT ( ) SI_UNIT ( $, .RADIAN. ) );
#8670=ORIENTED_EDGE ( 'NONE', *, *, #678, .T. ) ;
#8675=DIRECTION ( 'NONE',  ( 0.1453943818575021418, -0.000000000000000000, 0.9893737785712106714 ) ) ;
#8680=CARTESIAN_POINT ( 'NONE',  ( 9.375397774054407662, 3.000000000000000000, -11.70905276178460497 ) ) ;
#8682=CARTESIAN_POINT ( 'NONE',  ( -10.97318381393799136, 3.000000000000000000, -6.970598036433411693 ) ) ;
#8685=CARTESIAN_POINT ( 'NONE',  ( -14.82803603298502360, 3.000000000000000000, -2.264806262022826644 ) ) ;
#8698=CARTESIAN_POINT ( 'NONE',  ( 10.25006213149504752, 0.000000000000000000, -9.299128225235653744 ) ) ;
#8701=CARTESIAN_POINT ( 'NONE',  ( 5.741477348071313713, 0.000000000000000000, -13.86115248177180703 ) ) ;
#8704=CARTESIAN_POINT ( 'NONE',  ( 2.928250210355320959, 3.000000000000000000, -13.52637830886121506 ) ) ;
#8706=ORIENTED_EDGE ( 'NONE', *, *, #9107, .F. ) ;
#8711=CARTESIAN_POINT ( 'NONE',  ( -12.68816982652970893, 3.000000000000000000, 2.830255545554337004 ) ) ;
#8714=CARTESIAN_POINT ( 'NONE',  ( -0.1834773636644435324, 3.000000000000000000, -13.00394737445024873 ) ) ;
#8715=CARTESIAN_POINT ( 'NONE',  ( 30.73000000000000043, 3.000000000000000000, -3.999999999999999112 ) ) ;
#8727=PRESENTATION_STYLE_ASSIGNMENT (( #7573 ) ) ;
#8734=VERTEX_POINT ( 'NONE', #11427 ) ;
#8737=UNCERTAINTY_MEASURE_WITH_UNIT (LENGTH_MEASURE( 1.000000000000000082E-05 ), #9898, 'distance_accuracy_value', 'NONE');
#8740=CARTESIAN_POINT ( 'NONE',  ( -12.98835496148321944, 0.000000000000000000, -0.5501230721522551992 ) ) ;
#8745=CARTESIAN_POINT ( 'NONE',  ( 8.883544964651964193, 0.000000000000000000, -12.08646469655236544 ) ) ;
#8748=CARTESIAN_POINT ( 'NONE',  ( -7.500000000000000000, 0.000000000000000000, 1.500000000000000666 ) ) ;
#8751=VERTEX_POINT ( 'NONE', #8119 ) ;
#8755=EDGE_CURVE ( 'NONE', #6405, #13024, #2236, .T. ) ;
#8756=EDGE_CURVE ( 'NONE', #9161, #6340, #2717, .T. ) ;
#8758=DIRECTION ( 'NONE',  ( 0.000000000000000000, 1.000000000000000000, 0.000000000000000000 ) ) ;
#8761=CARTESIAN_POINT ( 'NONE',  ( -11.90284147956865723, 3.000000000000000000, -9.133371500908332052 ) ) ;
#8767=ADVANCED_FACE ( 'NONE', ( #9687 ), #3566, .F. ) ;
#8768=CARTESIAN_POINT ( 'NONE',  ( -5.452638258930639914, 3.000000000000000000, -13.97385902380748313 ) ) ;
#8773=CARTESIAN_POINT ( 'NONE',  ( 30.73000000000000043, 3.000000000000000000, -3.999999999999999112 ) ) ;
#8776=CARTESIAN_POINT ( 'NONE',  ( -10.97318381393799136, 3.000000000000000000, -6.970598036433411693 ) ) ;
#8794=CARTESIAN_POINT ( 'NONE',  ( -10.25006213149496936, 3.000000000000000000, -9.299128225235415712 ) ) ;
#8795=ORIENTED_EDGE ( 'NONE', *, *, #3563, .F. ) ;
#8799=CARTESIAN_POINT ( 'NONE',  ( -12.98835496148321944, 3.000000000000000000, -0.5501230721522551992 ) ) ;
#8804=CARTESIAN_POINT ( 'NONE',  ( -14.39763212228013955, 0.000000000000000000, -1.133238802859595884 ) ) ;
#8805=CARTESIAN_POINT ( 'NONE',  ( -12.30759122141990325, 0.000000000000000000, -6.329356821613475681 ) ) ;
#8807=CARTESIAN_POINT ( 'NONE',  ( -12.56843238770841786, 0.000000000000000000, 3.367671042046304741 ) ) ;
#8808=CARTESIAN_POINT ( 'NONE',  ( -14.20034848914876235, 3.000000000000000000, -2.631756770590732764 ) ) ;
#8814=ORIENTED_EDGE ( 'NONE', *, *, #11985, .F. ) ;
#8817=CARTESIAN_POINT ( 'NONE',  ( -14.90895795148411374, 3.000000000000000000, -1.650143266773683726 ) ) ;
#8826=CARTESIAN_POINT ( 'NONE',  ( 9.299128225235451239, 0.000000000000000000, -10.25006213149493561 ) ) ;
#8832=ORIENTED_EDGE ( 'NONE', *, *, #13393, .T. ) ;
#8843=CIRCLE ( 'NONE', #11064, 0.9999999999999997780 ) ;
#8847=CARTESIAN_POINT ( 'NONE',  ( -11.63517940784383775, 0.000000000000000000, -7.494008246337203083 ) ) ;
#8850=CARTESIAN_POINT ( 'NONE',  ( -12.40340517008309185, 3.000000000000000000, -3.893011711613028947 ) ) ;
#8851=ORIENTED_EDGE ( 'NONE', *, *, #11579, .T. ) ;
#8859=ORIENTED_EDGE ( 'NONE', *, *, #9113, .F. ) ;
#8868=B_SPLINE_CURVE_WITH_KNOTS ( 'NONE', 3,
 ( #13295, #11155, #11994, #10110 ),
 .UNSPECIFIED., .F., .F.,
 ( 4, 4 ),
 ( 0.09090310649439187207, 0.1203211835519651524 ),
 .UNSPECIFIED. ) ;
#8869=CARTESIAN_POINT ( 'NONE',  ( -11.52330688609014686, 0.000000000000000000, -6.017756925049552841 ) ) ;
#8872=CARTESIAN_POINT ( 'NONE',  ( 30.65246752842885058, 3.000000000000000000, -7.988606140548566437 ) ) ;
#8874=VERTEX_POINT ( 'NONE', #8850 ) ;
#8879=EDGE_CURVE ( 'NONE', #12419, #144, #461, .T. ) ;
#8887=CARTESIAN_POINT ( 'NONE',  ( -3.542894779577211661, 3.000000000000000000, -12.51336118825813948 ) ) ;
#8906=CARTESIAN_POINT ( 'NONE',  ( -9.065441275458884007, 0.000000000000000000, -9.324917484779556176 ) ) ;
#8916=B_SPLINE_SURFACE_WITH_KNOTS ( 'NONE', 3, 1, ( 
 ( #5188, #13527 ),
 ( #9387, #12561 ),
 ( #913, #6345 ),
 ( #4351, #9442 ) ),
 .UNSPECIFIED., .F., .F., .F.,
 ( 4, 4 ),
 ( 2, 2 ),
 ( 0.000000000000000000, 0.5855695330273008592 ),
 ( 0.000000000000000000, 1.000000000000000000 ),
 .UNSPECIFIED. ) ;
#8928=CARTESIAN_POINT ( 'NONE',  ( 11.90284147956858085, 3.000000000000000000, -9.133371500908429752 ) ) ;
#8930=ORIENTED_EDGE ( 'NONE', *, *, #13057, .F. ) ;
#8931=EDGE_CURVE ( 'NONE', #8734, #8874, #2898, .T. ) ;
#8937=B_SPLINE_CURVE_WITH_KNOTS ( 'NONE', 2,
 ( #3861, #2562, #10895 ),
 .UNSPECIFIED., .F., .F.,
 ( 3, 3 ),
 ( 0.000000000000000000, 1.000000000000000000 ),
 .UNSPECIFIED. ) ;
#8940=PLANE ( 'NONE',  #5614 ) ;
#8950=DIRECTION ( 'NONE',  ( 0.000000000000000000, 0.000000000000000000, -1.000000000000000000 ) ) ;
#8960=VERTEX_POINT ( 'NONE', #9140 ) ;
#8967=CARTESIAN_POINT ( 'NONE',  ( -8.883544964652065445, 0.000000000000000000, -12.08646469655229438 ) ) ;
#8969=LINE ( 'NONE', #438, #9894 ) ;
#8979=CARTESIAN_POINT ( 'NONE',  ( -6.660869762029062890, 0.000000000000000000, -11.17001010193236610 ) ) ;
#8990=CARTESIAN_POINT ( 'NONE',  ( -0.5501230721523990841, 0.000000000000000000, -12.98835496148299384 ) ) ;
#8995=EDGE_CURVE ( 'NONE', #7605, #11130, #3367, .T. ) ;
#8997=LINE ( 'NONE', #1722, #9689 ) ;
#9023=ORIENTED_EDGE ( 'NONE', *, *, #8879, .T. ) ;
#9035=CARTESIAN_POINT ( 'NONE',  ( -12.98835496148321944, 0.000000000000000000, -0.5501230721522551992 ) ) ;
#9047=ORIENTED_EDGE ( 'NONE', *, *, #11388, .F. ) ;
#9048=EDGE_LOOP ( 'NONE', ( #8063, #3002, #5688, #4958 ) ) ;
#9058=AXIS2_PLACEMENT_3D ( 'NONE', #2881, #3208, #11615 ) ;
#9059=CARTESIAN_POINT ( 'NONE',  ( 3.542895259386137585, 3.000000000000000000, -12.51336047125611017 ) ) ;
#9072=FACE_OUTER_BOUND ( 'NONE', #5328, .T. ) ;
#9076=EDGE_LOOP ( 'NONE', ( #11790, #449, #11665, #966 ) ) ;
#9083=ORIENTED_EDGE ( 'NONE', *, *, #9633, .F. ) ;
#9084=CARTESIAN_POINT ( 'NONE',  ( -14.87484884897978077, 3.000000000000000000, -1.958311002203079187 ) ) ;
#9088=CARTESIAN_POINT ( 'NONE',  ( 3.188443874008702661, 0.000000000000000000, -12.60833581801614578 ) ) ;
#9102=EDGE_LOOP ( 'NONE', ( #13139, #11483 ) ) ;
#9107=EDGE_CURVE ( 'NONE', #12419, #899, #5173, .T. ) ;
#9113=EDGE_CURVE ( 'NONE', #5803, #8184, #12300, .T. ) ;
#9114=CARTESIAN_POINT ( 'NONE',  ( 0.000000000000000000, 3.000000000000000000, 0.000000000000000000 ) ) ;
#9135=CARTESIAN_POINT ( 'NONE',  ( -11.70905276178463872, 0.000000000000000000, -9.375397774054366806 ) ) ;
#9136=CARTESIAN_POINT ( 'NONE',  ( -2.928250210355484828, 3.000000000000000000, -13.52637830886140335 ) ) ;
#9140=CARTESIAN_POINT ( 'NONE',  ( 11.70905276178455878, 0.000000000000000000, -9.375397774054460953 ) ) ;
#9142=ADVANCED_FACE ( 'NONE', ( #4840 ), #2706, .F. ) ;
#9155=ORIENTED_EDGE ( 'NONE', *, *, #10713, .T. ) ;
#9160=CARTESIAN_POINT ( 'NONE',  ( -2.928250210355484828, 3.000000000000000000, -13.52637830886140335 ) ) ;
#9161=VERTEX_POINT ( 'NONE', #10010 ) ;
#9164=CARTESIAN_POINT ( 'NONE',  ( -12.68816982652970893, 0.000000000000000000, 2.830255545554337004 ) ) ;
#9169=EDGE_CURVE ( 'NONE', #5374, #11838, #6871, .T. ) ;
#9183=CARTESIAN_POINT ( 'NONE',  ( -13.73660796332618261, 3.000000000000000000, -6.025412986832017204 ) ) ;
#9190=ADVANCED_FACE ( 'NONE', ( #2633 ), #10942, .F. ) ;
#9194=DIRECTION ( 'NONE',  ( 0.000000000000000000, 0.000000000000000000, 1.000000000000000000 ) ) ;
#9196=B_SPLINE_CURVE_WITH_KNOTS ( 'NONE', 3,
 ( #1771, #6109, #12396, #10248 ),
 .UNSPECIFIED., .F., .F.,
 ( 4, 4 ),
 ( 0.000000000000000000, 0.5855695330273008592 ),
 .UNSPECIFIED. ) ;
#9200=CARTESIAN_POINT ( 'NONE',  ( -2.264806262022998062, 0.000000000000000000, -14.82803603298499340 ) ) ;
#9205=LINE ( 'NONE', #4110, #8608 ) ;
#9208=CARTESIAN_POINT ( 'NONE',  ( -11.70905276178463872, 0.000000000000000000, -9.375397774054366806 ) ) ;
#9215=CARTESIAN_POINT ( 'NONE',  ( 30.79786191028635400, 3.000000000000000000, -6.999232361977355765 ) ) ;
#9220=CARTESIAN_POINT ( 'NONE',  ( -14.90895795148411374, 3.000000000000000000, -1.650143266773683726 ) ) ;
#9222=ORIENTED_EDGE ( 'NONE', *, *, #10057, .F. ) ;
#9228=VECTOR ( 'NONE', #12781, 1000.000000000000000 ) ;
#9231=CARTESIAN_POINT ( 'NONE',  ( 2.264806262022877714, 3.000000000000000000, -14.82803603298501471 ) ) ;
#9232=EDGE_LOOP ( 'NONE', ( #10440, #2010, #4484, #3119 ) ) ;
#9237=EDGE_LOOP ( 'NONE', ( #10101, #4503, #3121, #3632, #96, #11607, #4647, #4552, #8795, #11695, #13034, #3372, #13554, #12985, #10953, #9083, #13585, #5659, #10266, #11406, #11207, #8930, #8294, #10158, #6944, #4821, #557, #4224, #6795, #861, #12876, #4002, #5507, #9926, #10872, #11159, #3677, #1696, #10817, #6880, #6192, #1245, #161, #8490, #7661, #4349, #2303, #13107, #12518, #160, #10195, #11144, #13570, #6752 ) ) ;
#9247=CARTESIAN_POINT ( 'NONE',  ( -1.650143266773857142, 3.000000000000000000, -14.90895795148409952 ) ) ;
#9250=CARTESIAN_POINT ( 'NONE',  ( -9.573149624528719315, 3.000000000000000000, -8.795158114916407754 ) ) ;
#9251=VECTOR ( 'NONE', #5980, 1000.000000000000000 ) ;
#9256=VERTEX_POINT ( 'NONE', #4087 ) ;
#9275=EDGE_CURVE ( 'NONE', #13474, #8960, #10446, .T. ) ;
#9280=EDGE_CURVE ( 'NONE', #7515, #5524, #5495, .T. ) ;
#9284=LINE ( 'NONE', #6182, #10794 ) ;
#9288=B_SPLINE_CURVE_WITH_KNOTS ( 'NONE', 3,
 ( #1393, #228, #10632, #7720 ),
 .UNSPECIFIED., .F., .F.,
 ( 4, 4 ),
 ( 0.000000000000000000, 0.5855695330273008592 ),
 .UNSPECIFIED. ) ;
#9293=ORIENTED_EDGE ( 'NONE', *, *, #12054, .F. ) ;
#9305=CARTESIAN_POINT ( 'NONE',  ( -12.68816982652970893, 3.000000000000000000, 2.830255545554337004 ) ) ;
#9309=EDGE_LOOP ( 'NONE', ( #12021, #5662, #6260, #7211 ) ) ;
#9311=CARTESIAN_POINT ( 'NONE',  ( -6.025412986832177076, 0.000000000000000000, -13.73660796332610268 ) ) ;
#9318=AXIS2_PLACEMENT_3D ( 'NONE', #4616, #4824, #8950 ) ;
#9326=CARTESIAN_POINT ( 'NONE',  ( -9.375397774054503586, 3.000000000000000000, -11.70905276178452503 ) ) ;
#9328=CARTESIAN_POINT ( 'NONE',  ( -11.70905276178463872, 3.000000000000000000, -9.375397774054366806 ) ) ;
#9334=ORIENTED_EDGE ( 'NONE', *, *, #1366, .T. ) ;
#9335=ORIENTED_EDGE ( 'NONE', *, *, #10543, .F. ) ;
#9337=DIRECTION ( 'NONE',  ( -0.000000000000000000, -1.000000000000000000, -0.000000000000000000 ) ) ;
#9351=B_SPLINE_CURVE_WITH_KNOTS ( 'NONE', 3,
 ( #11326, #1895, #2988, #6984 ),
 .UNSPECIFIED., .F., .F.,
 ( 4, 4 ),
 ( 0.000000000000000000, 0.5855695330273008592 ),
 .UNSPECIFIED. ) ;
#9356=B_SPLINE_CURVE_WITH_KNOTS ( 'NONE', 3,
 ( #2262, #11776, #13573, #4129 ),
 .UNSPECIFIED., .F., .F.,
 ( 4, 4 ),
 ( 0.9090903094065657664, 0.9385083864668765097 ),
 .UNSPECIFIED. ) ;
#9371=ORIENTED_EDGE ( 'NONE', *, *, #5171, .T. ) ;
#9373=EDGE_CURVE ( 'NONE', #8874, #2998, #406, .T. ) ;
#9376=CARTESIAN_POINT ( 'NONE',  ( -1.650143266773857142, 0.000000000000000000, -14.90895795148409952 ) ) ;
#9379=DIRECTION ( 'NONE',  ( -0.000000000000000000, -1.000000000000000000, -0.000000000000000000 ) ) ;
#9387=CARTESIAN_POINT ( 'NONE',  ( -4.227250083625790467, 3.000000000000000000, -13.17831234185026013 ) ) ;
#9388=EDGE_CURVE ( 'NONE', #13098, #4297, #12960, .T. ) ;
#9397=DIRECTION ( 'NONE',  ( -0.000000000000000000, -1.000000000000000000, -0.000000000000000000 ) ) ;
#9405=EDGE_LOOP ( 'NONE', ( #4867, #1233, #3469, #12144 ) ) ;
#9408=CARTESIAN_POINT ( 'NONE',  ( 12.63269908545826503, 3.000000000000000000, -5.340493616518843467 ) ) ;
#9414=ORIENTED_EDGE ( 'NONE', *, *, #3292, .T. ) ;
#9426=CARTESIAN_POINT ( 'NONE',  ( -0.5501230721523990841, 0.000000000000000000, -12.98835496148299384 ) ) ;
#9432=CARTESIAN_POINT ( 'NONE',  ( -14.20034848914871795, 3.000000000000000000, 2.631756770590945482 ) ) ;
#9434=CARTESIAN_POINT ( 'NONE',  ( 0.6724118135762067183, 3.000000000000000000, -13.82336506795094344 ) ) ;
#9435=EDGE_CURVE ( 'NONE', #2998, #5225, #9288, .T. ) ;
#9437=CARTESIAN_POINT ( 'NONE',  ( -13.97385902380755240, 0.000000000000000000, -5.452638258930474713 ) ) ;
#9442=CARTESIAN_POINT ( 'NONE',  ( -5.452638258930639914, 0.000000000000000000, -13.97385902380748313 ) ) ;
#9445=CARTESIAN_POINT ( 'NONE',  ( 0.000000000000000000, 0.000000000000000000, 0.000000000000000000 ) ) ;
#9446=CARTESIAN_POINT ( 'NONE',  ( 9.573149624528804580, 0.000000000000000000, -8.795158114916638681 ) ) ;
#9458=EDGE_LOOP ( 'NONE', ( #6996, #11241 ) ) ;
#9478=EDGE_CURVE ( 'NONE', #2426, #2659, #9717, .T. ) ;
#9491=ORIENTED_EDGE ( 'NONE', *, *, #8319, .T. ) ;
#9499=B_SPLINE_SURFACE_WITH_KNOTS ( 'NONE', 3, 1, ( 
 ( #7116, #8326 ),
 ( #12553, #6134 ),
 ( #3096, #12289 ),
 ( #13517, #7185 ) ),
 .UNSPECIFIED., .F., .F., .F.,
 ( 4, 4 ),
 ( 2, 2 ),
 ( 0.000000000000000000, 0.5855695330273008592 ),
 ( 0.000000000000000000, 1.000000000000000000 ),
 .UNSPECIFIED. ) ;
#9500=CARTESIAN_POINT ( 'NONE',  ( -7.500000000000000000, 3.000000000000000000, -1.500000000000000666 ) ) ;
#9504=CARTESIAN_POINT ( 'NONE',  ( -13.61374091949023679, 0.000000000000000000, -4.821006024660923650 ) ) ;
#9509=VECTOR ( 'NONE', #5944, 1000.000000000000114 ) ;
#9518=DIRECTION ( 'NONE',  ( 0.000000000000000000, 1.000000000000000000, 0.000000000000000000 ) ) ;
#9520=LINE ( 'NONE', #990, #2317 ) ;
#9529=CARTESIAN_POINT ( 'NONE',  ( -8.795158114916672432, 3.000000000000000000, -9.573149624528774382 ) ) ;
#9536=VERTEX_POINT ( 'NONE', #8068 ) ;
#9542=LINE ( 'NONE', #6507, #2281 ) ;
#9552=VERTEX_POINT ( 'NONE', #4767 ) ;
#9553=CARTESIAN_POINT ( 'NONE',  ( 30.73000000000000043, 3.000000000000000000, -3.999999999999999112 ) ) ;
#9554=B_SPLINE_CURVE_WITH_KNOTS ( 'NONE', 3,
 ( #8817, #2631, #3728, #9928 ),
 .UNSPECIFIED., .F., .F.,
 ( 4, 4 ),
 ( 0.000000000000000000, 0.5855695330273008592 ),
 .UNSPECIFIED. ) ;
#9558=CARTESIAN_POINT ( 'NONE',  ( -12.40340517008309185, 0.000000000000000000, -3.893011711613028947 ) ) ;
#9570=VERTEX_POINT ( 'NONE', #699 ) ;
#9579=FACE_OUTER_BOUND ( 'NONE', #1308, .T. ) ;
#9589=CARTESIAN_POINT ( 'NONE',  ( -3.542894779577211661, 3.000000000000000000, -12.51336118825813948 ) ) ;
#9597=CARTESIAN_POINT ( 'NONE',  ( -14.90895795148409420, 0.000000000000000000, 1.650143266773909101 ) ) ;
#9598=ORIENTED_EDGE ( 'NONE', *, *, #8585, .T. ) ;
#9606=EDGE_CURVE ( 'NONE', #6828, #12771, #8619, .T. ) ;
#9613=ADVANCED_FACE ( 'NONE', ( #7995 ), #276, .F. ) ;
#9619=CARTESIAN_POINT ( 'NONE',  ( 6.970598036433451661, 3.000000000000000000, -10.97318381393796294 ) ) ;
#9626=DIRECTION ( 'NONE',  ( 0.000000000000000000, 1.000000000000000000, 0.000000000000000000 ) ) ;
#9632=EDGE_CURVE ( 'NONE', #12628, #12207, #8937, .T. ) ;
#9633=EDGE_CURVE ( 'NONE', #4532, #12628, #1385, .T. ) ;
#9635=( LENGTH_UNIT ( ) NAMED_UNIT ( * ) SI_UNIT ( .MILLI., .METRE. ) );
#9641=CARTESIAN_POINT ( 'NONE',  ( -13.17831234185052836, 0.000000000000000000, -4.227250083625696320 ) ) ;
#9650=CARTESIAN_POINT ( 'NONE',  ( 1.650143266773734796, 3.000000000000000000, -14.90895795148410841 ) ) ;
#9656=CARTESIAN_POINT ( 'NONE',  ( 2.830255545554135832, 3.000000000000000000, -12.68816982652952596 ) ) ;
#9666=DIRECTION ( 'NONE',  ( -0.000000000000000000, -1.000000000000000000, -0.000000000000000000 ) ) ;
#9670=CARTESIAN_POINT ( 'NONE',  ( -12.08646469655240097, 0.000000000000000000, -8.883544964651921561 ) ) ;
#9677=EDGE_CURVE ( 'NONE', #7207, #6405, #6978, .T. ) ;
#9681=VECTOR ( 'NONE', #838, 1000.000000000000000 ) ;
#9684=CARTESIAN_POINT ( 'NONE',  ( -12.08646469655240097, 3.000000000000000000, -8.883544964651921561 ) ) ;
#9685=CARTESIAN_POINT ( 'NONE',  ( -13.97385902380755240, 3.000000000000000000, -5.452638258930474713 ) ) ;
#9687=FACE_OUTER_BOUND ( 'NONE', #2889, .T. ) ;
#9689=VECTOR ( 'NONE', #13291, 1000.000000000000000 ) ;
#9702=CARTESIAN_POINT ( 'NONE',  ( 0.000000000000000000, 3.000000000000000000, -1.500000000000000222 ) ) ;
#9709=ORIENTED_EDGE ( 'NONE', *, *, #6232, .T. ) ;
#9710=ORIENTED_EDGE ( 'NONE', *, *, #4648, .F. ) ;
#9711=PLANE ( 'NONE',  #11274 ) ;
#9717=LINE ( 'NONE', #12832, #7320 ) ;
#9718=LINE ( 'NONE', #3311, #4620 ) ;
#9723=ORIENTED_EDGE ( 'NONE', *, *, #13083, .T. ) ;
#9725=B_SPLINE_SURFACE_WITH_KNOTS ( 'NONE', 3, 1, ( 
 ( #492, #11169 ),
 ( #4695, #6896 ),
 ( #8887, #3033 ),
 ( #10408, #11510 ) ),
 .UNSPECIFIED., .F., .F., .F.,
 ( 4, 4 ),
 ( 2, 2 ),
 ( 0.5454515525569062495, 0.5748696296145745510 ),
 ( 0.000000000000000000, 1.000000000000000000 ),
 .UNSPECIFIED. ) ;
#9733=CARTESIAN_POINT ( 'NONE',  ( -14.39763212228012534, 3.000000000000000000, 1.133238802859812155 ) ) ;
#9737=CARTESIAN_POINT ( 'NONE',  ( -12.68816982652953840, 0.000000000000000000, -2.830255545554093644 ) ) ;
#9740=VECTOR ( 'NONE', #4104, 1000.000000000000114 ) ;
#9753=CARTESIAN_POINT ( 'NONE',  ( -7.500000000000000000, 3.000000000000000000, 1.500000000000000666 ) ) ;
#9755=ADVANCED_FACE ( 'NONE', ( #1939 ), #1486, .F. ) ;
#9757=CARTESIAN_POINT ( 'NONE',  ( -7.500000000000000000, 3.000000000000000000, 0.000000000000000000 ) ) ;
#9763=VERTEX_POINT ( 'NONE', #10331 ) ;
#9765=ORIENTED_EDGE ( 'NONE', *, *, #4376, .T. ) ;
#9768=CIRCLE ( 'NONE', #13526, 0.9999999999999997780 ) ;
#9779=EDGE_CURVE ( 'NONE', #9763, #1814, #10581, .T. ) ;
#9784=ORIENTED_EDGE ( 'NONE', *, *, #10547, .T. ) ;
#9788=EDGE_CURVE ( 'NONE', #1110, #6430, #6229, .T. ) ;
#9789=CARTESIAN_POINT ( 'NONE',  ( 9.133371500908369356, 0.000000000000000000, -11.90284147956862171 ) ) ;
#9792=CIRCLE ( 'NONE', #8035, 1.499999999999997780 ) ;
#9814=EDGE_LOOP ( 'NONE', ( #524, #9335, #637, #2070 ) ) ;
#9818=CARTESIAN_POINT ( 'NONE',  ( -6.343077614891082128, 0.000000000000000000, -11.35348748332310720 ) ) ;
#9822=CARTESIAN_POINT ( 'NONE',  ( -12.08646469655240097, 0.000000000000000000, -8.883544964651921561 ) ) ;
#9832=SHAPE_REPRESENTATION_RELATIONSHIP ( 'NONE' , 'NONE' ,  #5135, #2434 ) ;
#9833=B_SPLINE_SURFACE_WITH_KNOTS ( 'NONE', 3, 1, ( 
 ( #2125, #3913 ),
 ( #4120, #8117 ),
 ( #7093, #5284 ),
 ( #10322, #1027 ) ),
 .UNSPECIFIED., .F., .F., .F.,
 ( 4, 4 ),
 ( 2, 2 ),
 ( 0.2727224849193458089, 0.3021405619770169415 ),
 ( 0.000000000000000000, 1.000000000000000000 ),
 .UNSPECIFIED. ) ;
#9837=CARTESIAN_POINT ( 'NONE',  ( -10.25006213149496936, 0.000000000000000000, -9.299128225235415712 ) ) ;
#9843=ADVANCED_FACE ( 'NONE', ( #3619 ), #10537, .F. ) ;
#9851=CARTESIAN_POINT ( 'NONE',  ( -14.90895795148411374, 0.000000000000000000, -1.650143266773683726 ) ) ;
#9854=CARTESIAN_POINT ( 'NONE',  ( -13.52637830886122572, 3.000000000000000000, -2.928250210355275218 ) ) ;
#9855=CARTESIAN_POINT ( 'NONE',  ( -12.98835496148299207, 0.000000000000000000, 0.5501230721524459355 ) ) ;
#9861=EDGE_CURVE ( 'NONE', #8751, #5374, #3479, .T. ) ;
#9867=CARTESIAN_POINT ( 'NONE',  ( -0.6724118135763151871, 3.000000000000000000, -13.82336506795071784 ) ) ;
#9876=EDGE_CURVE ( 'NONE', #9536, #12679, #7766, .T. ) ;
#9878=DIRECTION ( 'NONE',  ( -0.000000000000000000, -1.000000000000000000, -0.000000000000000000 ) ) ;
#9884=CARTESIAN_POINT ( 'NONE',  ( -6.970598036433426792, 3.000000000000000000, -10.97318381393771780 ) ) ;
#9885=CARTESIAN_POINT ( 'NONE',  ( -12.98835496148321944, 0.000000000000000000, -0.5501230721522551992 ) ) ;
#9893=CARTESIAN_POINT ( 'NONE',  ( -0.1834773636644435324, 3.000000000000000000, -13.00394737445024873 ) ) ;
#9894=VECTOR ( 'NONE', #6987, 1000.000000000000114 ) ;
#9896=VERTEX_POINT ( 'NONE', #1428 ) ;
#9898=( LENGTH_UNIT ( ) NAMED_UNIT ( * ) SI_UNIT ( .MILLI., .METRE. ) );
#9906=ORIENTED_EDGE ( 'NONE', *, *, #3167, .T. ) ;
#9909=ORIENTED_EDGE ( 'NONE', *, *, #8755, .T. ) ;
#9915=CARTESIAN_POINT ( 'NONE',  ( -12.98835496148321944, 0.000000000000000000, -0.5501230721522550882 ) ) ;
#9926=ORIENTED_EDGE ( 'NONE', *, *, #10284, .F. ) ;
#9928=CARTESIAN_POINT ( 'NONE',  ( -12.98835496148321944, 3.000000000000000000, -0.5501230721522551992 ) ) ;
#9932=CARTESIAN_POINT ( 'NONE',  ( 7.499999999999999112, 3.000000000000000000, 1.499999999999997780 ) ) ;
#9934=B_SPLINE_SURFACE_WITH_KNOTS ( 'NONE', 2, 1, ( 
 ( #2993, #7442 ),
 ( #12690, #10611 ),
 ( #9326, #4343 ) ),
 .UNSPECIFIED., .F., .F., .F.,
 ( 3, 3 ),
 ( 2, 2 ),
 ( 0.000000000000000000, 1.000000000000000000 ),
 ( 0.000000000000000000, 1.000000000000000000 ),
 .UNSPECIFIED. ) ;
#9955=ADVANCED_FACE ( 'NONE', ( #2859 ), #13036, .F. ) ;
#9957=DIRECTION ( 'NONE',  ( -0.000000000000000000, -1.000000000000000000, -0.000000000000000000 ) ) ;
#9961=ORIENTED_EDGE ( 'NONE', *, *, #3887, .T. ) ;
#9965=CIRCLE ( 'NONE', #11963, 1.500000000000000666 ) ;
#9966=CARTESIAN_POINT ( 'NONE',  ( 11.70905276178455878, 0.000000000000000000, -9.375397774054460953 ) ) ;
#9972=LINE ( 'NONE', #3494, #7286 ) ;
#9976=VECTOR ( 'NONE', #9379, 1000.000000000000000 ) ;
#9980=DIRECTION ( 'NONE',  ( -0.000000000000000000, -1.000000000000000000, -0.000000000000000000 ) ) ;
#9982=UNCERTAINTY_MEASURE_WITH_UNIT (LENGTH_MEASURE( 1.000000000000000082E-05 ), #4970, 'distance_accuracy_value', 'NONE');
#9991=CARTESIAN_POINT ( 'NONE',  ( -12.98835496148321944, 0.000000000000000000, -0.5501230721522551992 ) ) ;
#9997=VECTOR ( 'NONE', #12155, 1000.000000000000000 ) ;
#10001=VERTEX_POINT ( 'NONE', #1842 ) ;
#10007=AXIS2_PLACEMENT_3D ( 'NONE', #6754, #3381, #5712 ) ;
#10010=CARTESIAN_POINT ( 'NONE',  ( 30.73000000000000043, 0.000000000000000000, -2.499999999999995115 ) ) ;
#10020=EDGE_CURVE ( 'NONE', #899, #13387, #8110, .T. ) ;
#10026=CARTESIAN_POINT ( 'NONE',  ( -6.660869762029062890, 3.000000000000000000, -11.17001010193236610 ) ) ;
#10039=CARTESIAN_POINT ( 'NONE',  ( 0.5501230721522984979, 3.000000000000000000, -12.98835496148321766 ) ) ;
#10056=EDGE_CURVE ( 'NONE', #5504, #7515, #5335, .T. ) ;
#10057=EDGE_CURVE ( 'NONE', #8568, #13098, #13477, .T. ) ;
#10063=CARTESIAN_POINT ( 'NONE',  ( -6.217402469309367241, 0.000000000000000000, -13.03533457366727610 ) ) ;
#10069=VERTEX_POINT ( 'NONE', #8299 ) ;
#10080=CARTESIAN_POINT ( 'NONE',  ( 9.375397774054407662, 3.000000000000000000, -11.70905276178460497 ) ) ;
#10081=DIRECTION ( 'NONE',  ( -0.000000000000000000, -1.000000000000000000, -0.000000000000000000 ) ) ;
#10084=LINE ( 'NONE', #10152, #8407 ) ;
#10091=CARTESIAN_POINT ( 'NONE',  ( -14.90895795148409420, 3.000000000000000000, 1.650143266773909101 ) ) ;
#10101=ORIENTED_EDGE ( 'NONE', *, *, #11311, .F. ) ;
#10108=EDGE_CURVE ( 'NONE', #10501, #8960, #10576, .T. ) ;
#10109=DIRECTION ( 'NONE',  ( -0.000000000000000000, -1.000000000000000000, -0.000000000000000000 ) ) ;
#10110=CARTESIAN_POINT ( 'NONE',  ( -12.98835496148299207, 3.000000000000000000, 0.5501230721524459355 ) ) ;
#10124=ORIENTED_EDGE ( 'NONE', *, *, #12319, .F. ) ;
#10127=CARTESIAN_POINT ( 'NONE',  ( -6.025412986832177076, 3.000000000000000000, -13.73660796332610268 ) ) ;
#10141=B_SPLINE_CURVE_WITH_KNOTS ( 'NONE', 3,
 ( #3117, #12573, #7205, #7403 ),
 .UNSPECIFIED., .F., .F.,
 ( 4, 4 ),
 ( 0.2727224849193458089, 0.3021405619770169415 ),
 .UNSPECIFIED. ) ;
#10144=CARTESIAN_POINT ( 'NONE',  ( -8.180229652970899323, 3.000000000000000000, -11.90209577080756276 ) ) ;
#10152=CARTESIAN_POINT ( 'NONE',  ( 2.264806262022877714, 3.000000000000000000, -14.82803603298501471 ) ) ;
#10154=ORIENTED_EDGE ( 'NONE', *, *, #12666, .T. ) ;
#10158=ORIENTED_EDGE ( 'NONE', *, *, #8755, .F. ) ;
#10162=LINE ( 'NONE', #11200, #12103 ) ;
#10163=CARTESIAN_POINT ( 'NONE',  ( 0.000000000000000000, 3.000000000000000000, 0.000000000000000000 ) ) ;
#10171=EDGE_LOOP ( 'NONE', ( #13370, #881, #1570, #8291 ) ) ;
#10176=AXIS2_PLACEMENT_3D ( 'NONE', #5951, #1695, #12307 ) ;
#10191=ORIENTED_EDGE ( 'NONE', *, *, #9478, .T. ) ;
#10195=ORIENTED_EDGE ( 'NONE', *, *, #5471, .F. ) ;
#10196=CARTESIAN_POINT ( 'NONE',  ( -1.650143266773857142, 3.000000000000000000, -14.90895795148409952 ) ) ;
#10198=ORIENTED_EDGE ( 'NONE', *, *, #5471, .T. ) ;
#10200=FACE_OUTER_BOUND ( 'NONE', #606, .T. ) ;
#10207=EDGE_CURVE ( 'NONE', #4297, #746, #5569, .T. ) ;
#10213=CARTESIAN_POINT ( 'NONE',  ( 30.66173999750687784, 3.000000000000000000, 0.01003121477750366919 ) ) ;
#10217=VECTOR ( 'NONE', #5655, 1000.000000000000000 ) ;
#10227=CARTESIAN_POINT ( 'NONE',  ( -6.217402469309367241, 3.000000000000000000, -13.03533457366727610 ) ) ;
#10231=FACE_OUTER_BOUND ( 'NONE', #3611, .T. ) ;
#10242=CARTESIAN_POINT ( 'NONE',  ( 8.883544964651964193, 0.000000000000000000, -12.08646469655236544 ) ) ;
#10247=CIRCLE ( 'NONE', #8228, 1.000000000000000888 ) ;
#10248=CARTESIAN_POINT ( 'NONE',  ( -12.68816982652970893, 3.000000000000000000, 2.830255545554337004 ) ) ;
#10258=LINE ( 'NONE', #5221, #2519 ) ;
#10260=FACE_OUTER_BOUND ( 'NONE', #3612, .T. ) ;
#10262=CARTESIAN_POINT ( 'NONE',  ( 7.499999999999999112, 3.000000000000000000, 0.000000000000000000 ) ) ;
#10265=ORIENTED_EDGE ( 'NONE', *, *, #7592, .T. ) ;
#10266=ORIENTED_EDGE ( 'NONE', *, *, #2045, .F. ) ;
#10269=DIRECTION ( 'NONE',  ( 0.000000000000000000, 0.000000000000000000, -1.000000000000000000 ) ) ;
#10284=EDGE_CURVE ( 'NONE', #5247, #2130, #10409, .T. ) ;
#10304=CARTESIAN_POINT ( 'NONE',  ( 6.970598036433451661, 0.000000000000000000, -10.97318381393796294 ) ) ;
#10314=CARTESIAN_POINT ( 'NONE',  ( -2.830255545554292151, 0.000000000000000000, -12.68816982652971959 ) ) ;
#10319=CARTESIAN_POINT ( 'NONE',  ( 11.70905276178455878, 3.000000000000000000, -9.375397774054460953 ) ) ;
#10320=CARTESIAN_POINT ( 'NONE',  ( -11.70905276178463872, 3.000000000000000000, -9.375397774054366806 ) ) ;
#10322=CARTESIAN_POINT ( 'NONE',  ( -11.52330688609014686, 3.000000000000000000, -6.017756925049552841 ) ) ;
#10323=EDGE_CURVE ( 'NONE', #1441, #12311, #5462, .T. ) ;
#10327=CARTESIAN_POINT ( 'NONE',  ( 1.836970198721030181E-16, 3.000000000000000000, 1.500000000000000222 ) ) ;
#10331=CARTESIAN_POINT ( 'NONE',  ( -0.5501230721523990841, 0.000000000000000000, -12.98835496148299384 ) ) ;
#10337=CARTESIAN_POINT ( 'NONE',  ( 2.264806262022877714, 0.000000000000000000, -14.82803603298501471 ) ) ;
#10345=( GEOMETRIC_REPRESENTATION_CONTEXT ( 3 ) GLOBAL_UNCERTAINTY_ASSIGNED_CONTEXT ( ( #9982 ) ) GLOBAL_UNIT_ASSIGNED_CONTEXT ( ( #4970, #11312, #777 ) ) REPRESENTATION_CONTEXT ( 'NONE', 'WORKASPACE' ) );
#10357=EDGE_LOOP ( 'NONE', ( #8330, #11883 ) ) ;
#10369=EDGE_CURVE ( 'NONE', #9552, #6730, #6133, .T. ) ;
#10382=EDGE_CURVE ( 'NONE', #816, #8003, #5465, .T. ) ;
#10385=SHAPE_DEFINITION_REPRESENTATION ( #10608, #5135 ) ;
#10392=CARTESIAN_POINT ( 'NONE',  ( 12.48730470360076161, 3.000000000000000000, -6.329867395090054139 ) ) ;
#10401=B_SPLINE_SURFACE_WITH_KNOTS ( 'NONE', 2, 1, ( 
 ( #2563, #6757 ),
 ( #11168, #9789 ),
 ( #4558, #8745 ) ),
 .UNSPECIFIED., .F., .F., .F.,
 ( 3, 3 ),
 ( 2, 2 ),
 ( 0.000000000000000000, 1.000000000000000000 ),
 ( 0.000000000000000000, 1.000000000000000000 ),
 .UNSPECIFIED. ) ;
#10408=CARTESIAN_POINT ( 'NONE',  ( -3.893011711613112880, 3.000000000000000000, -12.40340517008282717 ) ) ;
#10409=B_SPLINE_CURVE_WITH_KNOTS ( 'NONE', 3,
 ( #317, #1271, #7613, #1480 ),
 .UNSPECIFIED., .F., .F.,
 ( 4, 4 ),
 ( 0.000000000000000000, 0.5855695330273008592 ),
 .UNSPECIFIED. ) ;
#10418=DIRECTION ( 'NONE',  ( 0.000000000000000000, 0.000000000000000000, 1.000000000000000000 ) ) ;
#10437=B_SPLINE_CURVE_WITH_KNOTS ( 'NONE', 3,
 ( #11305, #693, #12347, #1731 ),
 .UNSPECIFIED., .F., .F.,
 ( 4, 4 ),
 ( 0.000000000000000000, 0.5855695330273008592 ),
 .UNSPECIFIED. ) ;
#10440=ORIENTED_EDGE ( 'NONE', *, *, #13393, .F. ) ;
#10445=AXIS2_PLACEMENT_3D ( 'NONE', #7391, #9518, #6414 ) ;
#10446=B_SPLINE_CURVE_WITH_KNOTS ( 'NONE', 2,
 ( #7322, #13391, #4015 ),
 .UNSPECIFIED., .F., .F.,
 ( 3, 3 ),
 ( 0.000000000000000000, 1.000000000000000000 ),
 .UNSPECIFIED. ) ;
#10458=DIRECTION ( 'NONE',  ( 0.000000000000000000, 0.000000000000000000, 1.000000000000000000 ) ) ;
#10459=EDGE_CURVE ( 'NONE', #2448, #12983, #1040, .T. ) ;
#10464=CARTESIAN_POINT ( 'NONE',  ( 6.970598036433451661, 3.000000000000000000, -10.97318381393796294 ) ) ;
#10467=CARTESIAN_POINT ( 'NONE',  ( -12.40340517008309185, 3.000000000000000000, -3.893011711613028947 ) ) ;
#10473=ORIENTED_EDGE ( 'NONE', *, *, #5820, .F. ) ;
#10489=ORIENTED_EDGE ( 'NONE', *, *, #5656, .F. ) ;
#10496=CARTESIAN_POINT ( 'NONE',  ( 1.958311002203130480, 3.000000000000000000, -14.87484884897977366 ) ) ;
#10501=VERTEX_POINT ( 'NONE', #11396 ) ;
#10505=ADVANCED_FACE ( 'NONE', ( #4213 ), #10561, .T. ) ;
#10506=ORIENTED_EDGE ( 'NONE', *, *, #5308, .T. ) ;
#10510=CARTESIAN_POINT ( 'NONE',  ( 6.217402469309262436, 3.000000000000000000, -13.03533457366732939 ) ) ;
#10519=ORIENTED_EDGE ( 'NONE', *, *, #5202, .T. ) ;
#10522=CARTESIAN_POINT ( 'NONE',  ( 2.264806262022877714, 3.000000000000000000, -14.82803603298501471 ) ) ;
#10524=CARTESIAN_POINT ( 'NONE',  ( 8.883544964651964193, 3.000000000000000000, -12.08646469655236544 ) ) ;
#10530=CARTESIAN_POINT ( 'NONE',  ( 4.821006024660968947, 3.000000000000000000, -13.61374091949021015 ) ) ;
#10537=CYLINDRICAL_SURFACE ( 'NONE', #5779, 1.500000000000003997 ) ;
#10541=B_SPLINE_CURVE_WITH_KNOTS ( 'NONE', 3,
 ( #11763, #2329, #1285, #259 ),
 .UNSPECIFIED., .F., .F.,
 ( 4, 4 ),
 ( 0.4545418633443863987, 0.4839599404020549223 ),
 .UNSPECIFIED. ) ;
#10543=EDGE_CURVE ( 'NONE', #8003, #2891, #1958, .T. ) ;
#10546=ORIENTED_EDGE ( 'NONE', *, *, #5019, .T. ) ;
#10547=EDGE_CURVE ( 'NONE', #8350, #6828, #6766, .T. ) ;
#10551=ORIENTED_EDGE ( 'NONE', *, *, #11806, .T. ) ;
#10557=CARTESIAN_POINT ( 'NONE',  ( -9.375397774054503586, 3.000000000000000000, -11.70905276178452503 ) ) ;
#10559=CARTESIAN_POINT ( 'NONE',  ( -9.375397774054503586, 0.000000000000000000, -11.70905276178452503 ) ) ;
#10561=CYLINDRICAL_SURFACE ( 'NONE', #11299, 1.000000000000000888 ) ;
#10565=CARTESIAN_POINT ( 'NONE',  ( 8.883544964651964193, 3.000000000000000000, -12.08646469655236544 ) ) ;
#10567=ORIENTED_EDGE ( 'NONE', *, *, #5656, .T. ) ;
#10570=CIRCLE ( 'NONE', #2863, 12.99999999999977973 ) ;
#10576=LINE ( 'NONE', #1138, #12179 ) ;
#10581=B_SPLINE_CURVE_WITH_KNOTS ( 'NONE', 3,
 ( #13514, #8128, #12355, #9376 ),
 .UNSPECIFIED., .F., .F.,
 ( 4, 4 ),
 ( 0.000000000000000000, 0.5855695330273008592 ),
 .UNSPECIFIED. ) ;
#10596=CARTESIAN_POINT ( 'NONE',  ( 30.79786191028635400, 0.000000000000000000, -6.999232361977355765 ) ) ;
#10598=EDGE_LOOP ( 'NONE', ( #1382, #7466 ) ) ;
#10608=PRODUCT_DEFINITION_SHAPE ( 'NONE', 'NONE',  #11618 ) ;
#10611=CARTESIAN_POINT ( 'NONE',  ( -9.133371500908470608, 0.000000000000000000, -11.90284147956855065 ) ) ;
#10613=CARTESIAN_POINT ( 'NONE',  ( -13.61374091949023679, 3.000000000000000000, -4.821006024660923650 ) ) ;
#10620=ORIENTED_EDGE ( 'NONE', *, *, #13057, .T. ) ;
#10625=CARTESIAN_POINT ( 'NONE',  ( 0.6724118135762067183, 3.000000000000000000, -13.82336506795094344 ) ) ;
#10632=CARTESIAN_POINT ( 'NONE',  ( -14.20034848914876235, 3.000000000000000000, -2.631756770590732764 ) ) ;
#10635=CARTESIAN_POINT ( 'NONE',  ( -14.20034848914871795, 0.000000000000000000, 2.631756770590945482 ) ) ;
#10638=ORIENTED_EDGE ( 'NONE', *, *, #8995, .T. ) ;
#10640=ORIENTED_EDGE ( 'NONE', *, *, #10056, .F. ) ;
#10653=CARTESIAN_POINT ( 'NONE',  ( 7.499999999999999112, 3.000000000000000000, -1.499999999999997780 ) ) ;
#10656=ORIENTED_EDGE ( 'NONE', *, *, #4509, .T. ) ;
#10660=ADVANCED_FACE ( 'NONE', ( #10699, #300, #1467, #3248, #8545 ), #1258, .F. ) ;
#10661=AXIS2_PLACEMENT_3D ( 'NONE', #9757, #12934, #3483 ) ;
#10666=CARTESIAN_POINT ( 'NONE',  ( 6.025412986832064277, 3.000000000000000000, -13.73660796332615597 ) ) ;
#10669=CARTESIAN_POINT ( 'NONE',  ( -13.73660796332618261, 0.000000000000000000, -6.025412986832017204 ) ) ;
#10670=VECTOR ( 'NONE', #11171, 1000.000000000000000 ) ;
#10673=ORIENTED_EDGE ( 'NONE', *, *, #11103, .T. ) ;
#10674=ORIENTED_EDGE ( 'NONE', *, *, #2483, .T. ) ;
#10685=CARTESIAN_POINT ( 'NONE',  ( -13.61374091949023679, 0.000000000000000000, -4.821006024660923650 ) ) ;
#10690=ORIENTED_EDGE ( 'NONE', *, *, #6604, .F. ) ;
#10699=FACE_OUTER_BOUND ( 'NONE', #272, .T. ) ;
#10700=ADVANCED_FACE ( 'NONE', ( #6625 ), #6428, .F. ) ;
#10704=ORIENTED_EDGE ( 'NONE', *, *, #6528, .T. ) ;
#10705=DIRECTION ( 'NONE',  ( -0.000000000000000000, -1.000000000000000000, -0.000000000000000000 ) ) ;
#10708=EDGE_CURVE ( 'NONE', #8347, #6705, #11538, .T. ) ;
#10710=CARTESIAN_POINT ( 'NONE',  ( 0.5501230721522984979, 0.000000000000000000, -12.98835496148321766 ) ) ;
#10711=CARTESIAN_POINT ( 'NONE',  ( 6.025412986832064277, 0.000000000000000000, -13.73660796332615597 ) ) ;
#10713=EDGE_CURVE ( 'NONE', #5225, #8350, #6696, .T. ) ;
#10714=CARTESIAN_POINT ( 'NONE',  ( 6.025412986832064277, 3.000000000000000000, -13.73660796332615597 ) ) ;
#10720=EDGE_CURVE ( 'NONE', #2149, #868, #4560, .T. ) ;
#10729=CARTESIAN_POINT ( 'NONE',  ( 30.79786191028635400, 0.000000000000000000, -7.999232361977356653 ) ) ;
#10732=ORIENTED_EDGE ( 'NONE', *, *, #11810, .T. ) ;
#10741=EDGE_CURVE ( 'NONE', #6705, #916, #6281, .T. ) ;
#10749=ORIENTED_EDGE ( 'NONE', *, *, #5475, .T. ) ;
#10769=CARTESIAN_POINT ( 'NONE',  ( 7.499999999999999112, 3.000000000000000000, 1.499999999999997780 ) ) ;
#10770=PRODUCT_CONTEXT ( 'NONE', #10822, 'mechanical' ) ;
#10794=VECTOR ( 'NONE', #3769, 1000.000000000000000 ) ;
#10798=EDGE_CURVE ( 'NONE', #3116, #12311, #11696, .T. ) ;
#10817=ORIENTED_EDGE ( 'NONE', *, *, #5202, .F. ) ;
#10819=CARTESIAN_POINT ( 'NONE',  ( -14.39763212228013955, 3.000000000000000000, -1.133238802859595884 ) ) ;
#10822=APPLICATION_CONTEXT ( 'automotive_design' ) ;
#10826=CARTESIAN_POINT ( 'NONE',  ( 2.264806262022877714, 3.000000000000000000, -14.82803603298501471 ) ) ;
#10833=B_SPLINE_SURFACE_WITH_KNOTS ( 'NONE', 3, 1, ( 
 ( #1468, #5657 ),
 ( #9854, #423 ),
 ( #8808, #3589 ),
 ( #7793, #12011 ) ),
 .UNSPECIFIED., .F., .F., .F.,
 ( 4, 4 ),
 ( 2, 2 ),
 ( 0.000000000000000000, 0.5855695330273008592 ),
 ( 0.000000000000000000, 1.000000000000000000 ),
 .UNSPECIFIED. ) ;
#10834=B_SPLINE_CURVE_WITH_KNOTS ( 'NONE', 3,
 ( #13135, #9059, #3685, #2732 ),
 .UNSPECIFIED., .F., .F.,
 ( 4, 4 ),
 ( 0.7272709309819391787, 0.7566890080396341256 ),
 .UNSPECIFIED. ) ;
#10843=LINE ( 'NONE', #13114, #9997 ) ;
#10846=FACE_OUTER_BOUND ( 'NONE', #11381, .T. ) ;
#10847=LINE ( 'NONE', #1214, #13001 ) ;
#10852=ADVANCED_FACE ( 'NONE', ( #2689 ), #9725, .F. ) ;
#10856=CARTESIAN_POINT ( 'NONE',  ( -14.82803603298502360, 3.000000000000000000, -2.264806262022826644 ) ) ;
#10858=AXIS2_PLACEMENT_3D ( 'NONE', #3449, #7460, #4421 ) ;
#10866=CARTESIAN_POINT ( 'NONE',  ( 2.830255545554135832, 0.000000000000000000, -12.68816982652952596 ) ) ;
#10872=ORIENTED_EDGE ( 'NONE', *, *, #1288, .F. ) ;
#10881=CIRCLE ( 'NONE', #10445, 3.999999999999998224 ) ;
#10889=FACE_OUTER_BOUND ( 'NONE', #12384, .T. ) ;
#10890=ADVANCED_FACE ( 'NONE', ( #2007 ), #4565, .F. ) ;
#10891=VERTEX_POINT ( 'NONE', #4133 ) ;
#10893=B_SPLINE_CURVE_WITH_KNOTS ( 'NONE', 3,
 ( #10314, #1923, #3072, #13418 ),
 .UNSPECIFIED., .F., .F.,
 ( 4, 4 ),
 ( 0.5454515525569062495, 0.5748696296145745510 ),
 .UNSPECIFIED. ) ;
#10895=CARTESIAN_POINT ( 'NONE',  ( -13.97385902380755240, 0.000000000000000000, -5.452638258930474713 ) ) ;
#10903=ORIENTED_EDGE ( 'NONE', *, *, #565, .F. ) ;
#10907=EDGE_LOOP ( 'NONE', ( #9709, #12204, #10489, #1019 ) ) ;
#10912=CARTESIAN_POINT ( 'NONE',  ( 8.795158114916441505, 3.000000000000000000, -9.573149624528689117 ) ) ;
#10924=ADVANCED_FACE ( 'NONE', ( #8268 ), #6310, .F. ) ;
#10927=CARTESIAN_POINT ( 'NONE',  ( -10.97318381393799136, 3.000000000000000000, -6.970598036433411693 ) ) ;
#10931=ORIENTED_EDGE ( 'NONE', *, *, #7785, .F. ) ;
#10932=B_SPLINE_SURFACE_WITH_KNOTS ( 'NONE', 2, 1, ( 
 ( #3232, #1173 ),
 ( #1242, #8592 ),
 ( #6475, #215 ) ),
 .UNSPECIFIED., .F., .F., .F.,
 ( 3, 3 ),
 ( 2, 2 ),
 ( 0.000000000000000000, 1.000000000000000000 ),
 ( 0.000000000000000000, 1.000000000000000000 ),
 .UNSPECIFIED. ) ;
#10934=ORIENTED_EDGE ( 'NONE', *, *, #9779, .T. ) ;
#10938=EDGE_CURVE ( 'NONE', #10985, #11917, #6201, .T. ) ;
#10942=B_SPLINE_SURFACE_WITH_KNOTS ( 'NONE', 3, 1, ( 
 ( #6839, #5807 ),
 ( #4780, #1751 ),
 ( #10144, #3601 ),
 ( #4914, #8967 ) ),
 .UNSPECIFIED., .F., .F., .F.,
 ( 4, 4 ),
 ( 2, 2 ),
 ( 0.000000000000000000, 0.5855695330273008592 ),
 ( 0.000000000000000000, 1.000000000000000000 ),
 .UNSPECIFIED. ) ;
#10943=CARTESIAN_POINT ( 'NONE',  ( 12.63269908545826503, 0.000000000000000000, -5.340493616518841691 ) ) ;
#10949=CARTESIAN_POINT ( 'NONE',  ( -2.631756770590896632, 0.000000000000000000, -14.20034848914872505 ) ) ;
#10952=FACE_OUTER_BOUND ( 'NONE', #3253, .T. ) ;
#10953=ORIENTED_EDGE ( 'NONE', *, *, #9632, .F. ) ;
#10958=CARTESIAN_POINT ( 'NONE',  ( -6.017756925049793537, 0.000000000000000000, -11.52330688609026232 ) ) ;
#10970=ORIENTED_EDGE ( 'NONE', *, *, #4202, .T. ) ;
#10975=CARTESIAN_POINT ( 'NONE',  ( -1.133238802859761973, 0.000000000000000000, -14.39763212228013067 ) ) ;
#10978=CARTESIAN_POINT ( 'NONE',  ( 0.000000000000000000, 3.000000000000000000, 0.000000000000000000 ) ) ;
#10982=EDGE_LOOP ( 'NONE', ( #4396, #12079, #3898, #13204 ) ) ;
#10985=VERTEX_POINT ( 'NONE', #8525 ) ;
#10991=CARTESIAN_POINT ( 'NONE',  ( 6.660877044263387781, 0.000000000000000000, -11.16999893002129696 ) ) ;
#11012=VECTOR ( 'NONE', #11829, 1000.000000000000000 ) ;
#11013=DIRECTION ( 'NONE',  ( 0.000000000000000000, 0.000000000000000000, 1.000000000000000000 ) ) ;
#11014=ORIENTED_EDGE ( 'NONE', *, *, #12522, .T. ) ;
#11022=ORIENTED_EDGE ( 'NONE', *, *, #5820, .T. ) ;
#11041=CARTESIAN_POINT ( 'NONE',  ( 0.5501230721522984979, 3.000000000000000000, -12.98835496148321766 ) ) ;
#11042=CARTESIAN_POINT ( 'NONE',  ( -13.82336506795071607, 3.000000000000000000, 0.6724118135763649251 ) ) ;
#11052=ORIENTED_EDGE ( 'NONE', *, *, #7467, .T. ) ;
#11064=AXIS2_PLACEMENT_3D ( 'NONE', #11516, #8135, #8273 ) ;
#11066=CARTESIAN_POINT ( 'NONE',  ( 6.017756925049591921, 0.000000000000000000, -11.52330688609011844 ) ) ;
#11068=CARTESIAN_POINT ( 'NONE',  ( 3.893011711613070691, 0.000000000000000000, -12.40340517008307231 ) ) ;
#11070=CARTESIAN_POINT ( 'NONE',  ( -13.17831234185052836, 3.000000000000000000, -4.227250083625696320 ) ) ;
#11079=CYLINDRICAL_SURFACE ( 'NONE', #7470, 1.000000000000000888 ) ;
#11087=CARTESIAN_POINT ( 'NONE',  ( -5.452638258930639914, 3.000000000000000000, -13.97385902380748313 ) ) ;
#11092=ORIENTED_EDGE ( 'NONE', *, *, #8096, .T. ) ;
#11094=VERTEX_POINT ( 'NONE', #12812 ) ;
#11102=CARTESIAN_POINT ( 'NONE',  ( -6.970598036433426792, 3.000000000000000000, -10.97318381393771780 ) ) ;
#11103=EDGE_CURVE ( 'NONE', #916, #4831, #12199, .T. ) ;
#11104=CARTESIAN_POINT ( 'NONE',  ( -12.68816982652970893, 0.000000000000000000, 2.830255545554337004 ) ) ;
#11109=CARTESIAN_POINT ( 'NONE',  ( -13.73660796332618261, 3.000000000000000000, -6.025412986832017204 ) ) ;
#11130=VERTEX_POINT ( 'NONE', #9702 ) ;
#11132=CARTESIAN_POINT ( 'NONE',  ( -6.017756925049793537, 0.000000000000000000, -11.52330688609026232 ) ) ;
#11144=ORIENTED_EDGE ( 'NONE', *, *, #12666, .F. ) ;
#11155=CARTESIAN_POINT ( 'NONE',  ( -13.00394681030572208, 3.000000000000000000, -0.1834665838397169235 ) ) ;
#11159=ORIENTED_EDGE ( 'NONE', *, *, #12636, .F. ) ;
#11168=CARTESIAN_POINT ( 'NONE',  ( 9.133371500908369356, 3.000000000000000000, -11.90284147956862171 ) ) ;
#11169=CARTESIAN_POINT ( 'NONE',  ( -2.830255545554292151, 0.000000000000000000, -12.68816982652971959 ) ) ;
#11171=DIRECTION ( 'NONE',  ( -0.000000000000000000, -1.000000000000000000, -0.000000000000000000 ) ) ;
#11183=B_SPLINE_CURVE_WITH_KNOTS ( 'NONE', 3,
 ( #7591, #1190, #3307, #8680 ),
 .UNSPECIFIED., .F., .F.,
 ( 4, 4 ),
 ( 0.000000000000000000, 0.5855695330273008592 ),
 .UNSPECIFIED. ) ;
#11184=CARTESIAN_POINT ( 'NONE',  ( 3.893011711613070691, 3.000000000000000000, -12.40340517008307231 ) ) ;
#11187=CARTESIAN_POINT ( 'NONE',  ( -9.375397774054503586, 0.000000000000000000, -11.70905276178452503 ) ) ;
#11198=CARTESIAN_POINT ( 'NONE',  ( 12.63269908545826503, 3.000000000000000000, -5.340493616518841691 ) ) ;
#11199=CARTESIAN_POINT ( 'NONE',  ( -14.82803603298498629, 3.000000000000000000, 2.264806262023049577 ) ) ;
#11200=CARTESIAN_POINT ( 'NONE',  ( 9.375397774054407662, 3.000000000000000000, -11.70905276178460497 ) ) ;
#11201=FACE_OUTER_BOUND ( 'NONE', #10982, .T. ) ;
#11204=VERTEX_POINT ( 'NONE', #4751 ) ;
#11207=ORIENTED_EDGE ( 'NONE', *, *, #10369, .F. ) ;
#11208=DIRECTION ( 'NONE',  ( 0.000000000000000000, 0.000000000000000000, -1.000000000000000000 ) ) ;
#11216=CARTESIAN_POINT ( 'NONE',  ( 11.63517940784358196, 3.000000000000000000, -7.494008246337187096 ) ) ;
#11241=ORIENTED_EDGE ( 'NONE', *, *, #8756, .T. ) ;
#11249=VECTOR ( 'NONE', #7558, 1000.000000000000000 ) ;
#11258=CARTESIAN_POINT ( 'NONE',  ( 1.836970198721030181E-16, 0.000000000000000000, 1.500000000000000222 ) ) ;
#11262=VERTEX_POINT ( 'NONE', #7836 ) ;
#11269=CARTESIAN_POINT ( 'NONE',  ( -14.90895795148409420, 3.000000000000000000, 1.650143266773909101 ) ) ;
#11274=AXIS2_PLACEMENT_3D ( 'NONE', #4485, #8675, #2413 ) ;
#11281=CARTESIAN_POINT ( 'NONE',  ( 11.90284147956858085, 0.000000000000000000, -9.133371500908429752 ) ) ;
#11292=EDGE_CURVE ( 'NONE', #12227, #13024, #10258, .T. ) ;
#11293=DIRECTION ( 'NONE',  ( -0.000000000000000000, -1.000000000000000000, -0.000000000000000000 ) ) ;
#11297=VECTOR ( 'NONE', #9878, 1000.000000000000000 ) ;
#11298=DIRECTION ( 'NONE',  ( 0.000000000000000000, 0.000000000000000000, -1.000000000000000000 ) ) ;
#11299=AXIS2_PLACEMENT_3D ( 'NONE', #12449, #2025, #2921 ) ;
#11305=CARTESIAN_POINT ( 'NONE',  ( 6.017756925049591921, 3.000000000000000000, -11.52330688609011844 ) ) ;
#11310=DIRECTION ( 'NONE',  ( 0.000000000000000000, 0.000000000000000000, 1.000000000000000000 ) ) ;
#11311=EDGE_CURVE ( 'NONE', #10069, #3948, #9768, .T. ) ;
#11312=( NAMED_UNIT ( * ) PLANE_ANGLE_UNIT ( ) SI_UNIT ( $, .RADIAN. ) );
#11316=VERTEX_POINT ( 'NONE', #5017 ) ;
#11320=ORIENTED_EDGE ( 'NONE', *, *, #9388, .F. ) ;
#11324=ORIENTED_EDGE ( 'NONE', *, *, #1854, .T. ) ;
#11326=CARTESIAN_POINT ( 'NONE',  ( 11.70905276178455878, 3.000000000000000000, -9.375397774054460953 ) ) ;
#11331=VECTOR ( 'NONE', #4508, 1000.000000000000000 ) ;
#11340=VERTEX_POINT ( 'NONE', #13596 ) ;
#11354=VERTEX_POINT ( 'NONE', #5159 ) ;
#11364=CARTESIAN_POINT ( 'NONE',  ( 30.80713437936438126, 0.000000000000000000, 0.9994049933487144655 ) ) ;
#11365=CARTESIAN_POINT ( 'NONE',  ( 3.188443874008702661, 0.000000000000000000, -12.60833581801614578 ) ) ;
#11367=CARTESIAN_POINT ( 'NONE',  ( -12.51336114795298471, 0.000000000000000000, -3.542894103880322998 ) ) ;
#11369=ORIENTED_EDGE ( 'NONE', *, *, #1359, .T. ) ;
#11370=EDGE_LOOP ( 'NONE', ( #9906, #8814, #12848, #2753 ) ) ;
#11377=CARTESIAN_POINT ( 'NONE',  ( -12.40347894490204972, 3.000000000000000000, 3.892776652129660064 ) ) ;
#11381=EDGE_LOOP ( 'NONE', ( #10519, #7801, #2162, #10704 ) ) ;
#11388=EDGE_CURVE ( 'NONE', #10891, #5504, #8231, .T. ) ;
#11396=CARTESIAN_POINT ( 'NONE',  ( 11.70905276178455878, 3.000000000000000000, -9.375397774054460953 ) ) ;
#11399=LINE ( 'NONE', #1961, #12450 ) ;
#11402=VERTEX_POINT ( 'NONE', #4119 ) ;
#11403=EDGE_LOOP ( 'NONE', ( #9961, #1326, #7888, #6515 ) ) ;
#11406=ORIENTED_EDGE ( 'NONE', *, *, #3216, .F. ) ;
#11419=B_SPLINE_SURFACE_WITH_KNOTS ( 'NONE', 2, 1, ( 
 ( #2376, #3331 ),
 ( #8761, #2235 ),
 ( #11751, #9670 ) ),
 .UNSPECIFIED., .F., .F., .F.,
 ( 3, 3 ),
 ( 2, 2 ),
 ( 0.000000000000000000, 1.000000000000000000 ),
 ( 0.000000000000000000, 1.000000000000000000 ),
 .UNSPECIFIED. ) ;
#11420=VERTEX_POINT ( 'NONE', #10729 ) ;
#11426=CARTESIAN_POINT ( 'NONE',  ( -12.60833596047604210, 3.000000000000000000, -3.188441730140805674 ) ) ;
#11427=CARTESIAN_POINT ( 'NONE',  ( -13.97385902380755240, 3.000000000000000000, -5.452638258930474713 ) ) ;
#11428=EDGE_LOOP ( 'NONE', ( #11852, #10749, #6100, #5932 ) ) ;
#11436=CARTESIAN_POINT ( 'NONE',  ( 0.5501230721522984979, 3.000000000000000000, -12.98835496148321766 ) ) ;
#11442=ORIENTED_EDGE ( 'NONE', *, *, #10938, .F. ) ;
#11447=ORIENTED_EDGE ( 'NONE', *, *, #9107, .T. ) ;
#11464=EDGE_LOOP ( 'NONE', ( #2189, #3966, #11324, #4700 ) ) ;
#11466=EDGE_CURVE ( 'NONE', #11838, #5374, #11546, .T. ) ;
#11467=ORIENTED_EDGE ( 'NONE', *, *, #11292, .F. ) ;
#11470=B_SPLINE_CURVE_WITH_KNOTS ( 'NONE', 3,
 ( #11990, #2473, #3567, #757 ),
 .UNSPECIFIED., .F., .F.,
 ( 4, 4 ),
 ( 0.000000000000000000, 0.5855695330273008592 ),
 .UNSPECIFIED. ) ;
#11483=ORIENTED_EDGE ( 'NONE', *, *, #7416, .T. ) ;
#11488=CIRCLE ( 'NONE', #5755, 1.000000000000000888 ) ;
#11494=CARTESIAN_POINT ( 'NONE',  ( -14.20034848914876235, 0.000000000000000000, -2.631756770590732764 ) ) ;
#11498=VECTOR ( 'NONE', #3988, 1000.000000000000000 ) ;
#11502=VECTOR ( 'NONE', #8616, 1000.000000000000000 ) ;
#11510=CARTESIAN_POINT ( 'NONE',  ( -3.893011711613112880, 0.000000000000000000, -12.40340517008282717 ) ) ;
#11516=CARTESIAN_POINT ( 'NONE',  ( 30.80713437936438126, 3.000000000000000000, 0.9994049933487144655 ) ) ;
#11519=LINE ( 'NONE', #6750, #7740 ) ;
#11520=B_SPLINE_CURVE_WITH_KNOTS ( 'NONE', 3,
 ( #7957, #10991, #1769, #11066 ),
 .UNSPECIFIED., .F., .F.,
 ( 4, 4 ),
 ( 0.8181806201944104018, 0.8475986972523573693 ),
 .UNSPECIFIED. ) ;
#11523=VECTOR ( 'NONE', #8344, 1000.000000000000000 ) ;
#11525=CARTESIAN_POINT ( 'NONE',  ( -9.299128225235689271, 3.000000000000000000, -10.25006213149501555 ) ) ;
#11527=CARTESIAN_POINT ( 'NONE',  ( 1.650143266773734796, 3.000000000000000000, -14.90895795148410841 ) ) ;
#11530=CARTESIAN_POINT ( 'NONE',  ( 11.63517940784358196, 0.000000000000000000, -7.494008246337187096 ) ) ;
#11538=B_SPLINE_CURVE_WITH_KNOTS ( 'NONE', 3,
 ( #11932, #10635, #12765, #2495 ),
 .UNSPECIFIED., .F., .F.,
 ( 4, 4 ),
 ( 0.000000000000000000, 0.5855695330273008592 ),
 .UNSPECIFIED. ) ;
#11541=EDGE_CURVE ( 'NONE', #2998, #6481, #7560, .T. ) ;
#11546=CIRCLE ( 'NONE', #11974, 1.500000000000000666 ) ;
#11560=ADVANCED_FACE ( 'NONE', ( #8512 ), #4219, .F. ) ;
#11568=CIRCLE ( 'NONE', #7813, 1.499999999999997780 ) ;
#11574=CARTESIAN_POINT ( 'NONE',  ( 5.452638258930520010, 3.000000000000000000, -13.97385902380752754 ) ) ;
#11575=ORIENTED_EDGE ( 'NONE', *, *, #2045, .T. ) ;
#11579=EDGE_CURVE ( 'NONE', #3916, #12227, #5130, .T. ) ;
#11584=CARTESIAN_POINT ( 'NONE',  ( 1.133238802859644956, 0.000000000000000000, -14.39763212228013600 ) ) ;
#11590=ORIENTED_EDGE ( 'NONE', *, *, #4376, .F. ) ;
#11597=CARTESIAN_POINT ( 'NONE',  ( 9.065480927540312095, 0.000000000000000000, -9.324856600128422102 ) ) ;
#11607=ORIENTED_EDGE ( 'NONE', *, *, #10708, .F. ) ;
#11608=ORIENTED_EDGE ( 'NONE', *, *, #13322, .T. ) ;
#11615=DIRECTION ( 'NONE',  ( 0.000000000000000000, 0.000000000000000000, 1.000000000000000000 ) ) ;
#11618=PRODUCT_DEFINITION ( 'UNKNOWN', '', #1907, #3917 ) ;
#11625=CARTESIAN_POINT ( 'NONE',  ( 30.66173999750687784, 3.000000000000000000, 0.01003121477750366919 ) ) ;
#11632=CARTESIAN_POINT ( 'NONE',  ( 30.73000000000000043, 0.000000000000000000, -3.999999999999999112 ) ) ;
#11637=CARTESIAN_POINT ( 'NONE',  ( -1.650143266773857142, 0.000000000000000000, -14.90895795148409952 ) ) ;
#11638=ADVANCED_FACE ( 'NONE', ( #1433 ), #1370, .F. ) ;
#11651=ORIENTED_EDGE ( 'NONE', *, *, #1015, .T. ) ;
#11665=ORIENTED_EDGE ( 'NONE', *, *, #4725, .F. ) ;
#11666=LINE ( 'NONE', #6499, #2690 ) ;
#11670=CIRCLE ( 'NONE', #5715, 1.500000000000003997 ) ;
#11676=CARTESIAN_POINT ( 'NONE',  ( 11.70905276178455878, 3.000000000000000000, -9.375397774054460953 ) ) ;
#11677=FACE_OUTER_BOUND ( 'NONE', #42, .T. ) ;
#11679=CARTESIAN_POINT ( 'NONE',  ( -12.08646469655240097, 0.000000000000000000, -8.883544964651921561 ) ) ;
#11684=AXIS2_PLACEMENT_3D ( 'NONE', #10978, #6712, #7614 ) ;
#11687=B_SPLINE_CURVE_WITH_KNOTS ( 'NONE', 2,
 ( #11087, #7839, #556 ),
 .UNSPECIFIED., .F., .F.,
 ( 3, 3 ),
 ( 0.000000000000000000, 1.000000000000000000 ),
 .UNSPECIFIED. ) ;
#11695=ORIENTED_EDGE ( 'NONE', *, *, #9606, .F. ) ;
#11696=B_SPLINE_CURVE_WITH_KNOTS ( 'NONE', 3,
 ( #2765, #13030, #1529, #3790 ),
 .UNSPECIFIED., .F., .F.,
 ( 4, 4 ),
 ( 0.9090903094065657664, 0.9385083864668765097 ),
 .UNSPECIFIED. ) ;
#11706=CARTESIAN_POINT ( 'NONE',  ( 5.452638258930520010, 0.000000000000000000, -13.97385902380752754 ) ) ;
#11710=CARTESIAN_POINT ( 'NONE',  ( -6.017756925049793537, 0.000000000000000000, -11.52330688609026232 ) ) ;
#11711=CARTESIAN_POINT ( 'NONE',  ( -11.70905276178464050, 0.000000000000000000, -9.375397774054366806 ) ) ;
#11721=EDGE_LOOP ( 'NONE', ( #10620, #3442, #1661, #1197 ) ) ;
#11726=CARTESIAN_POINT ( 'NONE',  ( 9.325031192972383920, 0.000000000000000000, -9.065266643391169055 ) ) ;
#11729=CARTESIAN_POINT ( 'NONE',  ( -12.51336114795298471, 3.000000000000000000, -3.542894103880322998 ) ) ;
#11732=EDGE_CURVE ( 'NONE', #899, #2380, #11399, .T. ) ;
#11739=ORIENTED_EDGE ( 'NONE', *, *, #3867, .T. ) ;
#11744=ORIENTED_EDGE ( 'NONE', *, *, #2516, .F. ) ;
#11745=FACE_OUTER_BOUND ( 'NONE', #8157, .T. ) ;
#11750=CARTESIAN_POINT ( 'NONE',  ( 5.452638258930520010, 0.000000000000000000, -13.97385902380752754 ) ) ;
#11751=CARTESIAN_POINT ( 'NONE',  ( -12.08646469655240097, 3.000000000000000000, -8.883544964651921561 ) ) ;
#11763=CARTESIAN_POINT ( 'NONE',  ( -6.017756925049793537, 3.000000000000000000, -11.52330688609026232 ) ) ;
#11768=VECTOR ( 'NONE', #2284, 1000.000000000000114 ) ;
#11776=CARTESIAN_POINT ( 'NONE',  ( 9.325031192972383920, 3.000000000000000000, -9.065266643391169055 ) ) ;
#11782=B_SPLINE_CURVE_WITH_KNOTS ( 'NONE', 3,
 ( #6976, #7857, #7042, #13241 ),
 .UNSPECIFIED., .F., .F.,
 ( 4, 4 ),
 ( 0.000000000000000000, 0.5855695330273008592 ),
 .UNSPECIFIED. ) ;
#11790=ORIENTED_EDGE ( 'NONE', *, *, #935, .T. ) ;
#11791=DIRECTION ( 'NONE',  ( -0.000000000000000000, -1.000000000000000000, -0.000000000000000000 ) ) ;
#11793=ORIENTED_EDGE ( 'NONE', *, *, #12636, .T. ) ;
#11803=CARTESIAN_POINT ( 'NONE',  ( 6.343080161942737938, 3.000000000000000000, -11.35348358516942469 ) ) ;
#11805=ORIENTED_EDGE ( 'NONE', *, *, #5806, .F. ) ;
#11806=EDGE_CURVE ( 'NONE', #10001, #7949, #7594, .T. ) ;
#11810=EDGE_CURVE ( 'NONE', #10891, #4765, #5198, .T. ) ;
#11814=CARTESIAN_POINT ( 'NONE',  ( 6.217402469309262436, 0.000000000000000000, -13.03533457366732939 ) ) ;
#11816=CARTESIAN_POINT ( 'NONE',  ( 8.795158114916441505, 0.000000000000000000, -9.573149624528689117 ) ) ;
#11828=DIRECTION ( 'NONE',  ( -0.000000000000000000, -1.000000000000000000, -0.000000000000000000 ) ) ;
#11829=DIRECTION ( 'NONE',  ( -0.000000000000000000, -1.000000000000000000, -0.000000000000000000 ) ) ;
#11833=CARTESIAN_POINT ( 'NONE',  ( -13.73660796332618261, 0.000000000000000000, -6.025412986832017204 ) ) ;
#11836=ORIENTED_EDGE ( 'NONE', *, *, #12219, .T. ) ;
#11838=VERTEX_POINT ( 'NONE', #8748 ) ;
#11843=CARTESIAN_POINT ( 'NONE',  ( -6.025412986832177076, 0.000000000000000000, -13.73660796332610268 ) ) ;
#11852=ORIENTED_EDGE ( 'NONE', *, *, #1952, .T. ) ;
#11857=CARTESIAN_POINT ( 'NONE',  ( -13.73660796332618261, 3.000000000000000000, -6.025412986832017204 ) ) ;
#11864=CARTESIAN_POINT ( 'NONE',  ( -2.264806262022998062, 0.000000000000000000, -14.82803603298499340 ) ) ;
#11872=CARTESIAN_POINT ( 'NONE',  ( -14.82803603298498629, 3.000000000000000000, 2.264806262023049577 ) ) ;
#11879=EDGE_CURVE ( 'NONE', #144, #2380, #1176, .T. ) ;
#11883=ORIENTED_EDGE ( 'NONE', *, *, #9788, .F. ) ;
#11886=CARTESIAN_POINT ( 'NONE',  ( -14.87484884897978077, 3.000000000000000000, -1.958311002203079187 ) ) ;
#11917=VERTEX_POINT ( 'NONE', #11864 ) ;
#11919=VERTEX_POINT ( 'NONE', #12964 ) ;
#11932=CARTESIAN_POINT ( 'NONE',  ( -14.82803603298498629, 0.000000000000000000, 2.264806262023049577 ) ) ;
#11939=CARTESIAN_POINT ( 'NONE',  ( -6.017756925049793537, 3.000000000000000000, -11.52330688609026232 ) ) ;
#11940=B_SPLINE_SURFACE_WITH_KNOTS ( 'NONE', 3, 1, ( 
 ( #5372, #157 ),
 ( #8794, #9837 ),
 ( #13015, #7444 ),
 ( #4345, #11711 ) ),
 .UNSPECIFIED., .F., .F., .F.,
 ( 4, 4 ),
 ( 2, 2 ),
 ( 0.000000000000000000, 0.5855695330273008592 ),
 ( 0.000000000000000000, 1.000000000000000000 ),
 .UNSPECIFIED. ) ;
#11942=ORIENTED_EDGE ( 'NONE', *, *, #3629, .T. ) ;
#11948=CARTESIAN_POINT ( 'NONE',  ( 9.573149624528804580, 0.000000000000000000, -8.795158114916638681 ) ) ;
#11956=AXIS2_PLACEMENT_3D ( 'NONE', #7904, #9980, #13091 ) ;
#11957=ORIENTED_EDGE ( 'NONE', *, *, #2538, .T. ) ;
#11963=AXIS2_PLACEMENT_3D ( 'NONE', #5995, #64, #10458 ) ;
#11969=CARTESIAN_POINT ( 'NONE',  ( -11.90209577080766046, 3.000000000000000000, -8.180229652970757215 ) ) ;
#11974=AXIS2_PLACEMENT_3D ( 'NONE', #1228, #5354, #8574 ) ;
#11975=ORIENTED_EDGE ( 'NONE', *, *, #13471, .F. ) ;
#11985=EDGE_CURVE ( 'NONE', #2448, #1536, #3794, .T. ) ;
#11988=FILL_AREA_STYLE ('',( #1369 ) ) ;
#11990=CARTESIAN_POINT ( 'NONE',  ( -9.573149624528719315, 3.000000000000000000, -8.795158114916407754 ) ) ;
#11994=CARTESIAN_POINT ( 'NONE',  ( -13.00394572736061605, 3.000000000000000000, 0.1835083749157108701 ) ) ;
#12003=ORIENTED_EDGE ( 'NONE', *, *, #2980, .T. ) ;
#12004=CYLINDRICAL_SURFACE ( 'NONE', #9318, 0.9999999999999997780 ) ;
#12008=MECHANICAL_DESIGN_GEOMETRIC_PRESENTATION_REPRESENTATION('',(#7172),#2764);
#12011=CARTESIAN_POINT ( 'NONE',  ( -14.82803603298502360, 0.000000000000000000, -2.264806262022826644 ) ) ;
#12013=EDGE_LOOP ( 'NONE', ( #3724, #12971, #5920, #4966 ) ) ;
#12020=B_SPLINE_CURVE_WITH_KNOTS ( 'NONE', 3,
 ( #6545, #12748, #3433, #7644 ),
 .UNSPECIFIED., .F., .F.,
 ( 4, 4 ),
 ( 0.000000000000000000, 0.5855695330273008592 ),
 .UNSPECIFIED. ) ;
#12021=ORIENTED_EDGE ( 'NONE', *, *, #5398, .T. ) ;
#12025=CARTESIAN_POINT ( 'NONE',  ( -12.98835496148299207, 3.000000000000000000, 0.5501230721524459355 ) ) ;
#12026=CARTESIAN_POINT ( 'NONE',  ( -0.5501230721523990841, 3.000000000000000000, -12.98835496148299384 ) ) ;
#12029=CARTESIAN_POINT ( 'NONE',  ( -9.324917476840782982, 3.000000000000000000, -9.065441278446241924 ) ) ;
#12036=CARTESIAN_POINT ( 'NONE',  ( -14.87484884897975057, 0.000000000000000000, 1.958311002203303453 ) ) ;
#12042=CARTESIAN_POINT ( 'NONE',  ( -11.63517940784383775, 3.000000000000000000, -7.494008246337203083 ) ) ;
#12054=EDGE_CURVE ( 'NONE', #8874, #1651, #12218, .T. ) ;
#12056=DIRECTION ( 'NONE',  ( 0.000000000000000000, 1.000000000000000000, 0.000000000000000000 ) ) ;
#12058=ORIENTED_EDGE ( 'NONE', *, *, #11732, .F. ) ;
#12078=EDGE_CURVE ( 'NONE', #12207, #1651, #12677, .T. ) ;
#12079=ORIENTED_EDGE ( 'NONE', *, *, #4336, .F. ) ;
#12081=ORIENTED_EDGE ( 'NONE', *, *, #11541, .T. ) ;
#12085=DIRECTION ( 'NONE',  ( 0.000000000000000000, 1.000000000000000000, 0.000000000000000000 ) ) ;
#12086=EDGE_CURVE ( 'NONE', #5803, #3424, #7382, .T. ) ;
#12087=CARTESIAN_POINT ( 'NONE',  ( 30.82048254704846713, 3.000000000000000000, -7.998976482636475538 ) ) ;
#12103=VECTOR ( 'NONE', #2937, 1000.000000000000000 ) ;
#12104=LINE ( 'NONE', #9753, #11012 ) ;
#12126=CARTESIAN_POINT ( 'NONE',  ( -12.98835496148299207, 3.000000000000000000, 0.5501230721524459355 ) ) ;
#12142=CARTESIAN_POINT ( 'NONE',  ( -11.52330688609014686, 3.000000000000000000, -6.017756925049552841 ) ) ;
#12144=ORIENTED_EDGE ( 'NONE', *, *, #10056, .T. ) ;
#12154=ADVANCED_FACE ( 'NONE', ( #12434 ), #12926, .F. ) ;
#12155=DIRECTION ( 'NONE',  ( -0.000000000000000000, -1.000000000000000000, -0.000000000000000000 ) ) ;
#12162=CARTESIAN_POINT ( 'NONE',  ( -9.573149624528719315, 0.000000000000000000, -8.795158114916407754 ) ) ;
#12168=EDGE_LOOP ( 'NONE', ( #7636, #6632, #1309, #8670 ) ) ;
#12179=VECTOR ( 'NONE', #1974, 1000.000000000000000 ) ;
#12180=VECTOR ( 'NONE', #411, 1000.000000000000000 ) ;
#12197=CARTESIAN_POINT ( 'NONE',  ( 11.90209577080759296, 3.000000000000000000, -8.180229652970856691 ) ) ;
#12199=CIRCLE ( 'NONE', #8004, 12.99999999999977973 ) ;
#12204=ORIENTED_EDGE ( 'NONE', *, *, #7450, .F. ) ;
#12207=VERTEX_POINT ( 'NONE', #9437 ) ;
#12213=CARTESIAN_POINT ( 'NONE',  ( -6.017756925049793537, 3.000000000000000000, -11.52330688609026232 ) ) ;
#12215=B_SPLINE_CURVE_WITH_KNOTS ( 'NONE', 3,
 ( #5386, #34, #2290, #473 ),
 .UNSPECIFIED., .F., .F.,
 ( 4, 4 ),
 ( 0.8181806201944104018, 0.8475986972523573693 ),
 .UNSPECIFIED. ) ;
#12218=LINE ( 'NONE', #1741, #1654 ) ;
#12219=EDGE_CURVE ( 'NONE', #13401, #12534, #9792, .T. ) ;
#12224=ORIENTED_EDGE ( 'NONE', *, *, #10323, .T. ) ;
#12227=VERTEX_POINT ( 'NONE', #8529 ) ;
#12230=CARTESIAN_POINT ( 'NONE',  ( 12.08646469655232636, 0.000000000000000000, -8.883544964652022813 ) ) ;
#12231=DIRECTION ( 'NONE',  ( 0.000000000000000000, 0.000000000000000000, 1.000000000000000000 ) ) ;
#12233=DIRECTION ( 'NONE',  ( -0.000000000000000000, -1.000000000000000000, -0.000000000000000000 ) ) ;
#12246=ADVANCED_FACE ( 'NONE', ( #9579 ), #2135, .F. ) ;
#12254=EDGE_CURVE ( 'NONE', #3774, #2677, #5641, .T. ) ;
#12261=EDGE_CURVE ( 'NONE', #4567, #3774, #836, .T. ) ;
#12262=ORIENTED_EDGE ( 'NONE', *, *, #10108, .T. ) ;
#12277=EDGE_CURVE ( 'NONE', #7144, #13474, #12020, .T. ) ;
#12289=CARTESIAN_POINT ( 'NONE',  ( 9.379342464487701037, 0.000000000000000000, -10.98198414889939301 ) ) ;
#12291=ORIENTED_EDGE ( 'NONE', *, *, #7133, .T. ) ;
#12297=ADVANCED_FACE ( 'NONE', ( #6402 ), #11940, .F. ) ;
#12300=LINE ( 'NONE', #3730, #9509 ) ;
#12307=DIRECTION ( 'NONE',  ( 0.000000000000000000, 0.000000000000000000, -1.000000000000000000 ) ) ;
#12311=VERTEX_POINT ( 'NONE', #3295 ) ;
#12319=EDGE_CURVE ( 'NONE', #7860, #288, #11568, .T. ) ;
#12320=CARTESIAN_POINT ( 'NONE',  ( 12.57851281883977457, 0.000000000000000000, 3.283445639306028063 ) ) ;
#12328=ADVANCED_FACE ( 'NONE', ( #1582 ), #8940, .F. ) ;
#12332=EDGE_CURVE ( 'NONE', #11354, #12419, #8868, .T. ) ;
#12339=FACE_OUTER_BOUND ( 'NONE', #3060, .T. ) ;
#12347=CARTESIAN_POINT ( 'NONE',  ( 6.217402469309262436, 3.000000000000000000, -13.03533457366732939 ) ) ;
#12349=EDGE_CURVE ( 'NONE', #2149, #2448, #11687, .T. ) ;
#12351=VERTEX_POINT ( 'NONE', #6743 ) ;
#12355=CARTESIAN_POINT ( 'NONE',  ( -1.133238802859761973, 0.000000000000000000, -14.39763212228013067 ) ) ;
#12362=CARTESIAN_POINT ( 'NONE',  ( -14.82803603298502360, 0.000000000000000000, -2.264806262022826644 ) ) ;
#12379=CARTESIAN_POINT ( 'NONE',  ( 12.08646469655232636, 0.000000000000000000, -8.883544964652022813 ) ) ;
#12384=EDGE_LOOP ( 'NONE', ( #10198, #11320, #9222, #3262 ) ) ;
#12385=CIRCLE ( 'NONE', #8174, 3.999999999999998224 ) ;
#12388=DIRECTION ( 'NONE',  ( -0.000000000000000000, -1.000000000000000000, -0.000000000000000000 ) ) ;
#12395=CIRCLE ( 'NONE', #10176, 1.000000000000000888 ) ;
#12396=CARTESIAN_POINT ( 'NONE',  ( -13.52637830886139092, 3.000000000000000000, 2.928250210355532790 ) ) ;
#12401=CARTESIAN_POINT ( 'NONE',  ( -4.821006024661084410, 3.000000000000000000, -13.61374091949017640 ) ) ;
#12407=DIRECTION ( 'NONE',  ( 0.000000000000000000, 0.000000000000000000, 1.000000000000000000 ) ) ;
#12416=VECTOR ( 'NONE', #12388, 1000.000000000000000 ) ;
#12418=VECTOR ( 'NONE', #4638, 1000.000000000000000 ) ;
#12419=VERTEX_POINT ( 'NONE', #12126 ) ;
#12429=CARTESIAN_POINT ( 'NONE',  ( -6.970598036433426792, 0.000000000000000000, -10.97318381393771780 ) ) ;
#12434=FACE_OUTER_BOUND ( 'NONE', #2742, .T. ) ;
#12443=CARTESIAN_POINT ( 'NONE',  ( 2.830255545554135832, 3.000000000000000000, -12.68816982652952596 ) ) ;
#12445=CARTESIAN_POINT ( 'NONE',  ( -12.08646469655240097, 0.000000000000000000, -8.883544964651921561 ) ) ;
#12449=CARTESIAN_POINT ( 'NONE',  ( 30.79786191028635400, 3.000000000000000000, -6.999232361977355765 ) ) ;
#12450=VECTOR ( 'NONE', #6223, 1000.000000000000000 ) ;
#12451=EDGE_CURVE ( 'NONE', #6481, #8350, #522, .T. ) ;
#12452=CARTESIAN_POINT ( 'NONE',  ( -7.500000000000000000, 0.000000000000000000, -1.500000000000000666 ) ) ;
#12454=ADVANCED_FACE ( 'NONE', ( #12339 ), #9833, .F. ) ;
#12465=LINE ( 'NONE', #12524, #12416 ) ;
#12469=CARTESIAN_POINT ( 'NONE',  ( 0.000000000000000000, 3.000000000000000000, 0.000000000000000000 ) ) ;
#12471=DIRECTION ( 'NONE',  ( 0.000000000000000000, 1.000000000000000000, 0.000000000000000000 ) ) ;
#12495=ADVANCED_FACE ( 'NONE', ( #10260 ), #5323, .F. ) ;
#12496=CARTESIAN_POINT ( 'NONE',  ( -8.795158114916672432, 0.000000000000000000, -9.573149624528774382 ) ) ;
#12497=EDGE_CURVE ( 'NONE', #13098, #4042, #2318, .T. ) ;
#12498=CARTESIAN_POINT ( 'NONE',  ( 10.97318381393774089, 0.000000000000000000, -6.970598036433387712 ) ) ;
#12513=ADVANCED_FACE ( 'NONE', ( #8379 ), #8255, .T. ) ;
#12514=CARTESIAN_POINT ( 'NONE',  ( 11.90209577080759296, 0.000000000000000000, -8.180229652970856691 ) ) ;
#12518=ORIENTED_EDGE ( 'NONE', *, *, #3887, .F. ) ;
#12522=EDGE_CURVE ( 'NONE', #1110, #9161, #7364, .T. ) ;
#12524=CARTESIAN_POINT ( 'NONE',  ( -12.40347894490204972, 3.000000000000000000, 3.892776652129660064 ) ) ;
#12534=VERTEX_POINT ( 'NONE', #4328 ) ;
#12538=CARTESIAN_POINT ( 'NONE',  ( 10.25006213149504752, 0.000000000000000000, -9.299128225235653744 ) ) ;
#12540=CARTESIAN_POINT ( 'NONE',  ( -12.68816982652953840, 0.000000000000000000, -2.830255545554093644 ) ) ;
#12542=ORIENTED_EDGE ( 'NONE', *, *, #866, .T. ) ;
#12543=EDGE_CURVE ( 'NONE', #11130, #3210, #73, .T. ) ;
#12548=CARTESIAN_POINT ( 'NONE',  ( -12.68816982652953840, 3.000000000000000000, -2.830255545554093644 ) ) ;
#12549=CARTESIAN_POINT ( 'NONE',  ( 30.73000000000000043, 3.000000000000000000, -3.999999999999999112 ) ) ;
#12553=CARTESIAN_POINT ( 'NONE',  ( 9.299128225235451239, 3.000000000000000000, -10.25006213149493561 ) ) ;
#12561=CARTESIAN_POINT ( 'NONE',  ( -4.227250083625790467, 0.000000000000000000, -13.17831234185026013 ) ) ;
#12567=DIRECTION ( 'NONE',  ( -0.000000000000000000, -1.000000000000000000, -0.000000000000000000 ) ) ;
#12568=CARTESIAN_POINT ( 'NONE',  ( -10.97318381393799136, 0.000000000000000000, -6.970598036433411693 ) ) ;
#12573=CARTESIAN_POINT ( 'NONE',  ( -11.17001009226120445, 3.000000000000000000, -6.660869730750943241 ) ) ;
#12604=CARTESIAN_POINT ( 'NONE',  ( -12.68816982652953840, 0.000000000000000000, -2.830255545554093644 ) ) ;
#12606=CARTESIAN_POINT ( 'NONE',  ( -2.928250210355484828, 0.000000000000000000, -13.52637830886140335 ) ) ;
#12611=AXIS2_PLACEMENT_3D ( 'NONE', #12549, #7110, #11310 ) ;
#12616=CARTESIAN_POINT ( 'NONE',  ( 3.893011711613070691, 0.000000000000000000, -12.40340517008307231 ) ) ;
#12618=CARTESIAN_POINT ( 'NONE',  ( -9.379342464487789854, 0.000000000000000000, -10.98198414889931307 ) ) ;
#12628=VERTEX_POINT ( 'NONE', #11833 ) ;
#12633=CARTESIAN_POINT ( 'NONE',  ( 9.325031192972383920, 3.000000000000000000, -9.065266643391169055 ) ) ;
#12636=EDGE_CURVE ( 'NONE', #2659, #11402, #12976, .T. ) ;
#12650=VECTOR ( 'NONE', #6317, 1000.000000000000000 ) ;
#12655=DIRECTION ( 'NONE',  ( -0.000000000000000000, -1.000000000000000000, -0.000000000000000000 ) ) ;
#12659=ORIENTED_EDGE ( 'NONE', *, *, #4582, .T. ) ;
#12666=EDGE_CURVE ( 'NONE', #11420, #4097, #10247, .T. ) ;
#12677=B_SPLINE_CURVE_WITH_KNOTS ( 'NONE', 3,
 ( #908, #9504, #5179, #13518 ),
 .UNSPECIFIED., .F., .F.,
 ( 4, 4 ),
 ( 0.000000000000000000, 0.5855695330273008592 ),
 .UNSPECIFIED. ) ;
#12679=VERTEX_POINT ( 'NONE', #6527 ) ;
#12684=ADVANCED_FACE ( 'NONE', ( #263 ), #4454, .F. ) ;
#12690=CARTESIAN_POINT ( 'NONE',  ( -9.133371500908470608, 3.000000000000000000, -11.90284147956855065 ) ) ;
#12692=LINE ( 'NONE', #156, #1355 ) ;
#12699=ORIENTED_EDGE ( 'NONE', *, *, #11806, .F. ) ;
#12700=CARTESIAN_POINT ( 'NONE',  ( 0.5501230721522984979, 3.000000000000000000, -12.98835496148321766 ) ) ;
#12701=CARTESIAN_POINT ( 'NONE',  ( 12.63269908545826503, 3.000000000000000000, -5.340493616518841691 ) ) ;
#12714=CARTESIAN_POINT ( 'NONE',  ( -14.39763212228012534, 0.000000000000000000, 1.133238802859812155 ) ) ;
#12716=CARTESIAN_POINT ( 'NONE',  ( 12.08646469655232636, 3.000000000000000000, -8.883544964652022813 ) ) ;
#12719=VERTEX_POINT ( 'NONE', #604 ) ;
#12726=CARTESIAN_POINT ( 'NONE',  ( -12.40347894490204794, 0.000000000000000000, 3.892776652129663173 ) ) ;
#12729=FACE_OUTER_BOUND ( 'NONE', #13385, .T. ) ;
#12734=CARTESIAN_POINT ( 'NONE',  ( 4.821006024660968947, 0.000000000000000000, -13.61374091949021015 ) ) ;
#12738=ORIENTED_EDGE ( 'NONE', *, *, #857, .T. ) ;
#12742=EDGE_CURVE ( 'NONE', #8751, #6867, #3835, .T. ) ;
#12748=CARTESIAN_POINT ( 'NONE',  ( 11.63517940784358196, 0.000000000000000000, -7.494008246337187096 ) ) ;
#12749=VERTEX_POINT ( 'NONE', #11068 ) ;
#12758=LINE ( 'NONE', #1117, #11768 ) ;
#12765=CARTESIAN_POINT ( 'NONE',  ( -13.52637830886139092, 0.000000000000000000, 2.928250210355532790 ) ) ;
#12771=VERTEX_POINT ( 'NONE', #9885 ) ;
#12774=VECTOR ( 'NONE', #10081, 1000.000000000000000 ) ;
#12781=DIRECTION ( 'NONE',  ( -0.000000000000000000, -1.000000000000000000, -0.000000000000000000 ) ) ;
#12789=B_SPLINE_CURVE_WITH_KNOTS ( 'NONE', 2,
 ( #6491, #4210, #10559 ),
 .UNSPECIFIED., .F., .F.,
 ( 3, 3 ),
 ( 0.000000000000000000, 1.000000000000000000 ),
 .UNSPECIFIED. ) ;
#12804=ORIENTED_EDGE ( 'NONE', *, *, #9113, .T. ) ;
#12812=CARTESIAN_POINT ( 'NONE',  ( -9.375397774054503586, 3.000000000000000000, -11.70905276178452503 ) ) ;
#12815=DIRECTION ( 'NONE',  ( 0.000000000000000000, 1.000000000000000000, 0.000000000000000000 ) ) ;
#12818=EDGE_CURVE ( 'NONE', #5500, #2426, #10834, .T. ) ;
#12832=CARTESIAN_POINT ( 'NONE',  ( 2.830255545554135832, 3.000000000000000000, -12.68816982652952596 ) ) ;
#12836=CARTESIAN_POINT ( 'NONE',  ( 2.631756770590782057, 3.000000000000000000, -14.20034848914875347 ) ) ;
#12840=CARTESIAN_POINT ( 'NONE',  ( 6.660877044263387781, 3.000000000000000000, -11.16999893002129696 ) ) ;
#12848=ORIENTED_EDGE ( 'NONE', *, *, #12349, .F. ) ;
#12852=EDGE_CURVE ( 'NONE', #13387, #12719, #9196, .T. ) ;
#12855=CARTESIAN_POINT ( 'NONE',  ( -2.264806262022998062, 3.000000000000000000, -14.82803603298499340 ) ) ;
#12864=CARTESIAN_POINT ( 'NONE',  ( 8.883544964651964193, 3.000000000000000000, -12.08646469655236544 ) ) ;
#12865=CARTESIAN_POINT ( 'NONE',  ( -13.73660796332618261, 3.000000000000000000, -6.025412986832017204 ) ) ;
#12866=B_SPLINE_CURVE_WITH_KNOTS ( 'NONE', 3,
 ( #5050, #1830, #3944, #9247 ),
 .UNSPECIFIED., .F., .F.,
 ( 4, 4 ),
 ( 0.000000000000000000, 0.5855695330273008592 ),
 .UNSPECIFIED. ) ;
#12868=CYLINDRICAL_SURFACE ( 'NONE', #3749, 1.500000000000003997 ) ;
#12871=VECTOR ( 'NONE', #1883, 1000.000000000000000 ) ;
#12874=CARTESIAN_POINT ( 'NONE',  ( -6.970598036433426792, 0.000000000000000000, -10.97318381393771780 ) ) ;
#12876=ORIENTED_EDGE ( 'NONE', *, *, #1015, .F. ) ;
#12882=EDGE_LOOP ( 'NONE', ( #10970, #11014, #6900, #7763 ) ) ;
#12899=ORIENTED_EDGE ( 'NONE', *, *, #9388, .T. ) ;
#12901=DIRECTION ( 'NONE',  ( -0.000000000000000000, -1.000000000000000000, -0.000000000000000000 ) ) ;
#12909=CARTESIAN_POINT ( 'NONE',  ( 6.017756925049591921, 0.000000000000000000, -11.52330688609011844 ) ) ;
#12910=ORIENTED_EDGE ( 'NONE', *, *, #6353, .T. ) ;
#12920=CARTESIAN_POINT ( 'NONE',  ( 2.264806262022877714, 3.000000000000000000, -14.82803603298501471 ) ) ;
#12923=ADVANCED_FACE ( 'NONE', ( #8163 ), #5661, .F. ) ;
#12925=EDGE_CURVE ( 'NONE', #2380, #8347, #1314, .T. ) ;
#12926=B_SPLINE_SURFACE_WITH_KNOTS ( 'NONE', 2, 1, ( 
 ( #9231, #10337 ),
 ( #8270, #6339 ),
 ( #2079, #3997 ) ),
 .UNSPECIFIED., .F., .F., .F.,
 ( 3, 3 ),
 ( 2, 2 ),
 ( 0.000000000000000000, 1.000000000000000000 ),
 ( 0.000000000000000000, 1.000000000000000000 ),
 .UNSPECIFIED. ) ;
#12928=CARTESIAN_POINT ( 'NONE',  ( -12.68816982652970893, 0.000000000000000000, 2.830255545554337004 ) ) ;
#12932=CARTESIAN_POINT ( 'NONE',  ( -11.63517940784383775, 3.000000000000000000, -7.494008246337203083 ) ) ;
#12934=DIRECTION ( 'NONE',  ( -0.000000000000000000, -1.000000000000000000, -0.000000000000000000 ) ) ;
#12955=CARTESIAN_POINT ( 'NONE',  ( -12.98835496148299207, 3.000000000000000000, 0.5501230721524460465 ) ) ;
#12960=LINE ( 'NONE', #12701, #5548 ) ;
#12964=CARTESIAN_POINT ( 'NONE',  ( -3.893011711613112880, 3.000000000000000000, -12.40340517008282717 ) ) ;
#12971=ORIENTED_EDGE ( 'NONE', *, *, #3714, .F. ) ;
#12976=B_SPLINE_CURVE_WITH_KNOTS ( 'NONE', 3,
 ( #10866, #4254, #1356, #2251 ),
 .UNSPECIFIED., .F., .F.,
 ( 4, 4 ),
 ( 0.000000000000000000, 0.5855695330273008592 ),
 .UNSPECIFIED. ) ;
#12978=CARTESIAN_POINT ( 'NONE',  ( 5.452638258930520010, 3.000000000000000000, -13.97385902380752754 ) ) ;
#12983=VERTEX_POINT ( 'NONE', #2523 ) ;
#12985=ORIENTED_EDGE ( 'NONE', *, *, #12078, .F. ) ;
#12989=LINE ( 'NONE', #4727, #11297 ) ;
#12993=DIRECTION ( 'NONE',  ( 0.000000000000000000, 0.000000000000000000, -1.000000000000000000 ) ) ;
#13000=ORIENTED_EDGE ( 'NONE', *, *, #1948, .T. ) ;
#13001=VECTOR ( 'NONE', #1416, 1000.000000000000000 ) ;
#13015=CARTESIAN_POINT ( 'NONE',  ( -10.98198414889942676, 3.000000000000000000, -9.379342464487661957 ) ) ;
#13018=EDGE_LOOP ( 'NONE', ( #10934, #1762, #2412, #1837 ) ) ;
#13023=CIRCLE ( 'NONE', #9058, 1.500000000000000222 ) ;
#13024=VERTEX_POINT ( 'NONE', #13129 ) ;
#13028=CARTESIAN_POINT ( 'NONE',  ( 30.79170750349150509, 0.000000000000000000, -0.0004760053210284623249 ) ) ;
#13030=CARTESIAN_POINT ( 'NONE',  ( 9.325031192972383920, 0.000000000000000000, -9.065266643391169055 ) ) ;
#13034=ORIENTED_EDGE ( 'NONE', *, *, #10547, .F. ) ;
#13036=B_SPLINE_SURFACE_WITH_KNOTS ( 'NONE', 2, 1, ( 
 ( #11269, #3892 ),
 ( #1916, #2794 ),
 ( #3958, #7003 ) ),
 .UNSPECIFIED., .F., .F., .F.,
 ( 3, 3 ),
 ( 2, 2 ),
 ( 0.000000000000000000, 1.000000000000000000 ),
 ( 0.000000000000000000, 1.000000000000000000 ),
 .UNSPECIFIED. ) ;
#13050=CARTESIAN_POINT ( 'NONE',  ( 9.379342464487701037, 0.000000000000000000, -10.98198414889939301 ) ) ;
#13057=EDGE_CURVE ( 'NONE', #5187, #9552, #4584, .T. ) ;
#13068=CARTESIAN_POINT ( 'NONE',  ( -10.97318381393799136, 0.000000000000000000, -6.970598036433411693 ) ) ;
#13071=CARTESIAN_POINT ( 'NONE',  ( -13.97385902380755240, 3.000000000000000000, -5.452638258930474713 ) ) ;
#13083=EDGE_CURVE ( 'NONE', #2891, #6390, #2298, .T. ) ;
#13091=DIRECTION ( 'NONE',  ( 0.000000000000000000, 0.000000000000000000, -1.000000000000000000 ) ) ;
#13095=CARTESIAN_POINT ( 'NONE',  ( 1.650143266773734796, 3.000000000000000000, -14.90895795148410841 ) ) ;
#13098=VERTEX_POINT ( 'NONE', #11198 ) ;
#13104=CARTESIAN_POINT ( 'NONE',  ( -12.40347894490204972, 0.000000000000000000, 3.892776652129660064 ) ) ;
#13107=ORIENTED_EDGE ( 'NONE', *, *, #12277, .F. ) ;
#13110=ORIENTED_EDGE ( 'NONE', *, *, #678, .F. ) ;
#13114=CARTESIAN_POINT ( 'NONE',  ( 30.79786191028635400, 3.000000000000000000, -7.999232361977356653 ) ) ;
#13129=CARTESIAN_POINT ( 'NONE',  ( -8.883544964652065445, 0.000000000000000000, -12.08646469655229438 ) ) ;
#13135=CARTESIAN_POINT ( 'NONE',  ( 3.893011711613070691, 3.000000000000000000, -12.40340517008307231 ) ) ;
#13139=ORIENTED_EDGE ( 'NONE', *, *, #2578, .T. ) ;
#13140=ORIENTED_EDGE ( 'NONE', *, *, #12852, .T. ) ;
#13141=FACE_OUTER_BOUND ( 'NONE', #9076, .T. ) ;
#13152=CARTESIAN_POINT ( 'NONE',  ( -11.35348746973813761, 0.000000000000000000, -6.343077501554963860 ) ) ;
#13162=B_SPLINE_CURVE_WITH_KNOTS ( 'NONE', 3,
 ( #9650, #1051, #10625, #12700 ),
 .UNSPECIFIED., .F., .F.,
 ( 4, 4 ),
 ( 0.000000000000000000, 0.5855695330273008592 ),
 .UNSPECIFIED. ) ;
#13165=CARTESIAN_POINT ( 'NONE',  ( -12.30759122141990325, 3.000000000000000000, -6.329356821613475681 ) ) ;
#13171=ORIENTED_EDGE ( 'NONE', *, *, #7422, .F. ) ;
#13180=CARTESIAN_POINT ( 'NONE',  ( -12.60833596047604210, 0.000000000000000000, -3.188441730140805674 ) ) ;
#13182=ADVANCED_FACE ( 'NONE', ( #8625 ), #499, .F. ) ;
#13193=CARTESIAN_POINT ( 'NONE',  ( -6.970598036433426792, 3.000000000000000000, -10.97318381393771780 ) ) ;
#13197=CYLINDRICAL_SURFACE ( 'NONE', #696, 12.99999999999977973 ) ;
#13204=ORIENTED_EDGE ( 'NONE', *, *, #10938, .T. ) ;
#13216=CARTESIAN_POINT ( 'NONE',  ( 0.000000000000000000, 0.000000000000000000, 0.000000000000000000 ) ) ;
#13233=CARTESIAN_POINT ( 'NONE',  ( -6.329356821613726147, 0.000000000000000000, -12.30759122142001338 ) ) ;
#13238=LINE ( 'NONE', #12142, #5977 ) ;
#13241=CARTESIAN_POINT ( 'NONE',  ( -6.017756925049793537, 0.000000000000000000, -11.52330688609026232 ) ) ;
#13253=CARTESIAN_POINT ( 'NONE',  ( -7.500000000000000000, 0.000000000000000000, 0.000000000000000000 ) ) ;
#13254=CARTESIAN_POINT ( 'NONE',  ( -13.00394572736061605, 0.000000000000000000, 0.1835083749157108701 ) ) ;
#13263=ORIENTED_EDGE ( 'NONE', *, *, #5046, .T. ) ;
#13267=EDGE_CURVE ( 'NONE', #8960, #3116, #165, .T. ) ;
#13270=CARTESIAN_POINT ( 'NONE',  ( 8.180229652970799847, 0.000000000000000000, -11.90209577080762848 ) ) ;
#13287=ORIENTED_EDGE ( 'NONE', *, *, #4427, .F. ) ;
#13291=DIRECTION ( 'NONE',  ( -0.000000000000000000, -1.000000000000000000, -0.000000000000000000 ) ) ;
#13294=DIRECTION ( 'NONE',  ( 0.000000000000000000, 0.000000000000000000, -1.000000000000000000 ) ) ;
#13295=CARTESIAN_POINT ( 'NONE',  ( -12.98835496148321944, 3.000000000000000000, -0.5501230721522551992 ) ) ;
#13305=CARTESIAN_POINT ( 'NONE',  ( 2.830255545554135832, 0.000000000000000000, -12.68816982652952596 ) ) ;
#13322=EDGE_CURVE ( 'NONE', #1608, #1814, #315, .T. ) ;
#13323=EDGE_CURVE ( 'NONE', #4042, #3324, #6483, .T. ) ;
#13337=LINE ( 'NONE', #1693, #1787 ) ;
#13350=FACE_OUTER_BOUND ( 'NONE', #9237, .T. ) ;
#13351=DIRECTION ( 'NONE',  ( 0.000000000000000000, 0.000000000000000000, -1.000000000000000000 ) ) ;
#13362=CARTESIAN_POINT ( 'NONE',  ( 10.97318381393774089, 3.000000000000000000, -6.970598036433387712 ) ) ;
#13370=ORIENTED_EDGE ( 'NONE', *, *, #9606, .T. ) ;
#13375=CARTESIAN_POINT ( 'NONE',  ( 8.883544964651964193, 0.000000000000000000, -12.08646469655236544 ) ) ;
#13377=CARTESIAN_POINT ( 'NONE',  ( -12.68816982652970893, 3.000000000000000000, 2.830255545554337004 ) ) ;
#13382=ORIENTED_EDGE ( 'NONE', *, *, #6763, .F. ) ;
#13385=EDGE_LOOP ( 'NONE', ( #9723, #7492, #2550, #3157 ) ) ;
#13387=VERTEX_POINT ( 'NONE', #11872 ) ;
#13391=CARTESIAN_POINT ( 'NONE',  ( 11.90284147956858085, 0.000000000000000000, -9.133371500908429752 ) ) ;
#13393=EDGE_CURVE ( 'NONE', #9896, #11420, #10843, .T. ) ;
#13396=CARTESIAN_POINT ( 'NONE',  ( 5.741477348071313713, 0.000000000000000000, -13.86115248177180703 ) ) ;
#13399=DIRECTION ( 'NONE',  ( -0.000000000000000000, -1.000000000000000000, -0.000000000000000000 ) ) ;
#13401=VERTEX_POINT ( 'NONE', #10769 ) ;
#13402=ORIENTED_EDGE ( 'NONE', *, *, #448, .T. ) ;
#13403=VERTEX_POINT ( 'NONE', #11041 ) ;
#13405=CARTESIAN_POINT ( 'NONE',  ( -9.379342464487789854, 0.000000000000000000, -10.98198414889931307 ) ) ;
#13408=FACE_BOUND ( 'NONE', #9458, .T. ) ;
#13409=CARTESIAN_POINT ( 'NONE',  ( -2.631756770590896632, 0.000000000000000000, -14.20034848914872505 ) ) ;
#13412=AXIS2_PLACEMENT_3D ( 'NONE', #3904, #3973, #12407 ) ;
#13418=CARTESIAN_POINT ( 'NONE',  ( -3.893011711613112880, 0.000000000000000000, -12.40340517008282717 ) ) ;
#13427=DIRECTION ( 'NONE',  ( 0.000000000000000000, 0.000000000000000000, -1.000000000000000000 ) ) ;
#13428=VERTEX_POINT ( 'NONE', #4984 ) ;
#13430=AXIS2_PLACEMENT_3D ( 'NONE', #2267, #4402, #2343 ) ;
#13432=MECHANICAL_DESIGN_GEOMETRIC_PRESENTATION_REPRESENTATION('',(#5288),#10345);
#13435=CARTESIAN_POINT ( 'NONE',  ( -12.40347894490204972, 0.000000000000000000, 3.892776652129660064 ) ) ;
#13445=CARTESIAN_POINT ( 'NONE',  ( -9.299128225235689271, 0.000000000000000000, -10.25006213149501555 ) ) ;
#13466=CYLINDRICAL_SURFACE ( 'NONE', #5095, 1.000000000000001776 ) ;
#13471=EDGE_CURVE ( 'NONE', #10501, #6263, #9351, .T. ) ;
#13474=VERTEX_POINT ( 'NONE', #12230 ) ;
#13475=CARTESIAN_POINT ( 'NONE',  ( -3.893011711613112880, 3.000000000000000000, -12.40340517008282717 ) ) ;
#13477=LINE ( 'NONE', #9408, #9740 ) ;
#13478=DIRECTION ( 'NONE',  ( 0.000000000000000000, -1.000000000000000000, 0.000000000000000000 ) ) ;
#13484=ORIENTED_EDGE ( 'NONE', *, *, #6113, .T. ) ;
#13498=DIRECTION ( 'NONE',  ( -0.000000000000000000, -1.000000000000000000, 0.000000000000000000 ) ) ;
#13502=AXIS2_PLACEMENT_3D ( 'NONE', #8358, #7276, #8495 ) ;
#13510=CARTESIAN_POINT ( 'NONE',  ( 30.73000000000000043, 3.000000000000000000, -3.999999999999999112 ) ) ;
#13514=CARTESIAN_POINT ( 'NONE',  ( -0.5501230721523990841, 0.000000000000000000, -12.98835496148299384 ) ) ;
#13517=CARTESIAN_POINT ( 'NONE',  ( 9.375397774054407662, 3.000000000000000000, -11.70905276178460497 ) ) ;
#13518=CARTESIAN_POINT ( 'NONE',  ( -12.40340517008309185, 0.000000000000000000, -3.893011711613028947 ) ) ;
#13520=CARTESIAN_POINT ( 'NONE',  ( -14.82803603298498629, 0.000000000000000000, 2.264806262023049577 ) ) ;
#13526=AXIS2_PLACEMENT_3D ( 'NONE', #11364, #5982, #6186 ) ;
#13527=CARTESIAN_POINT ( 'NONE',  ( -3.893011711613112880, 0.000000000000000000, -12.40340517008282717 ) ) ;
#13529=CARTESIAN_POINT ( 'NONE',  ( 1.650143266773734796, 3.000000000000000000, -14.90895795148410841 ) ) ;
#13534=CARTESIAN_POINT ( 'NONE',  ( 8.883544964651964193, 3.000000000000000000, -12.08646469655236544 ) ) ;
#13537=CARTESIAN_POINT ( 'NONE',  ( -9.573149624528719315, 0.000000000000000000, -8.795158114916407754 ) ) ;
#13542=ORIENTED_EDGE ( 'NONE', *, *, #4899, .F. ) ;
#13545=ORIENTED_EDGE ( 'NONE', *, *, #448, .F. ) ;
#13551=EDGE_CURVE ( 'NONE', #4042, #746, #9520, .T. ) ;
#13554=ORIENTED_EDGE ( 'NONE', *, *, #5506, .F. ) ;
#13570=ORIENTED_EDGE ( 'NONE', *, *, #1269, .F. ) ;
#13573=CARTESIAN_POINT ( 'NONE',  ( 9.065480927540312095, 3.000000000000000000, -9.324856600128422102 ) ) ;
#13575=ADVANCED_FACE ( 'NONE', ( #6284 ), #1147, .F. ) ;
#13582=EDGE_CURVE ( 'NONE', #11262, #6390, #5249, .T. ) ;
#13585=ORIENTED_EDGE ( 'NONE', *, *, #7363, .F. ) ;
#13596=CARTESIAN_POINT ( 'NONE',  ( -2.830255545554292151, 0.000000000000000000, -12.68816982652971959 ) ) ;
#13657=COLOUR_RGB('Off White',0.89,0.88,0.83);
#13658=FILL_AREA_STYLE_COLOUR('',#13657);
#13659=FILL_AREA_STYLE('',(#13658));
#13660=SURFACE_STYLE_FILL_AREA(#13659);
#13661=SURFACE_SIDE_STYLE('',(#13660));
#13662=SURFACE_STYLE_USAGE(.BOTH.,#13661);
#13663=PRESENTATION_STYLE_ASSIGNMENT((#13662));
ENDSEC;
END-ISO-10303-21;
